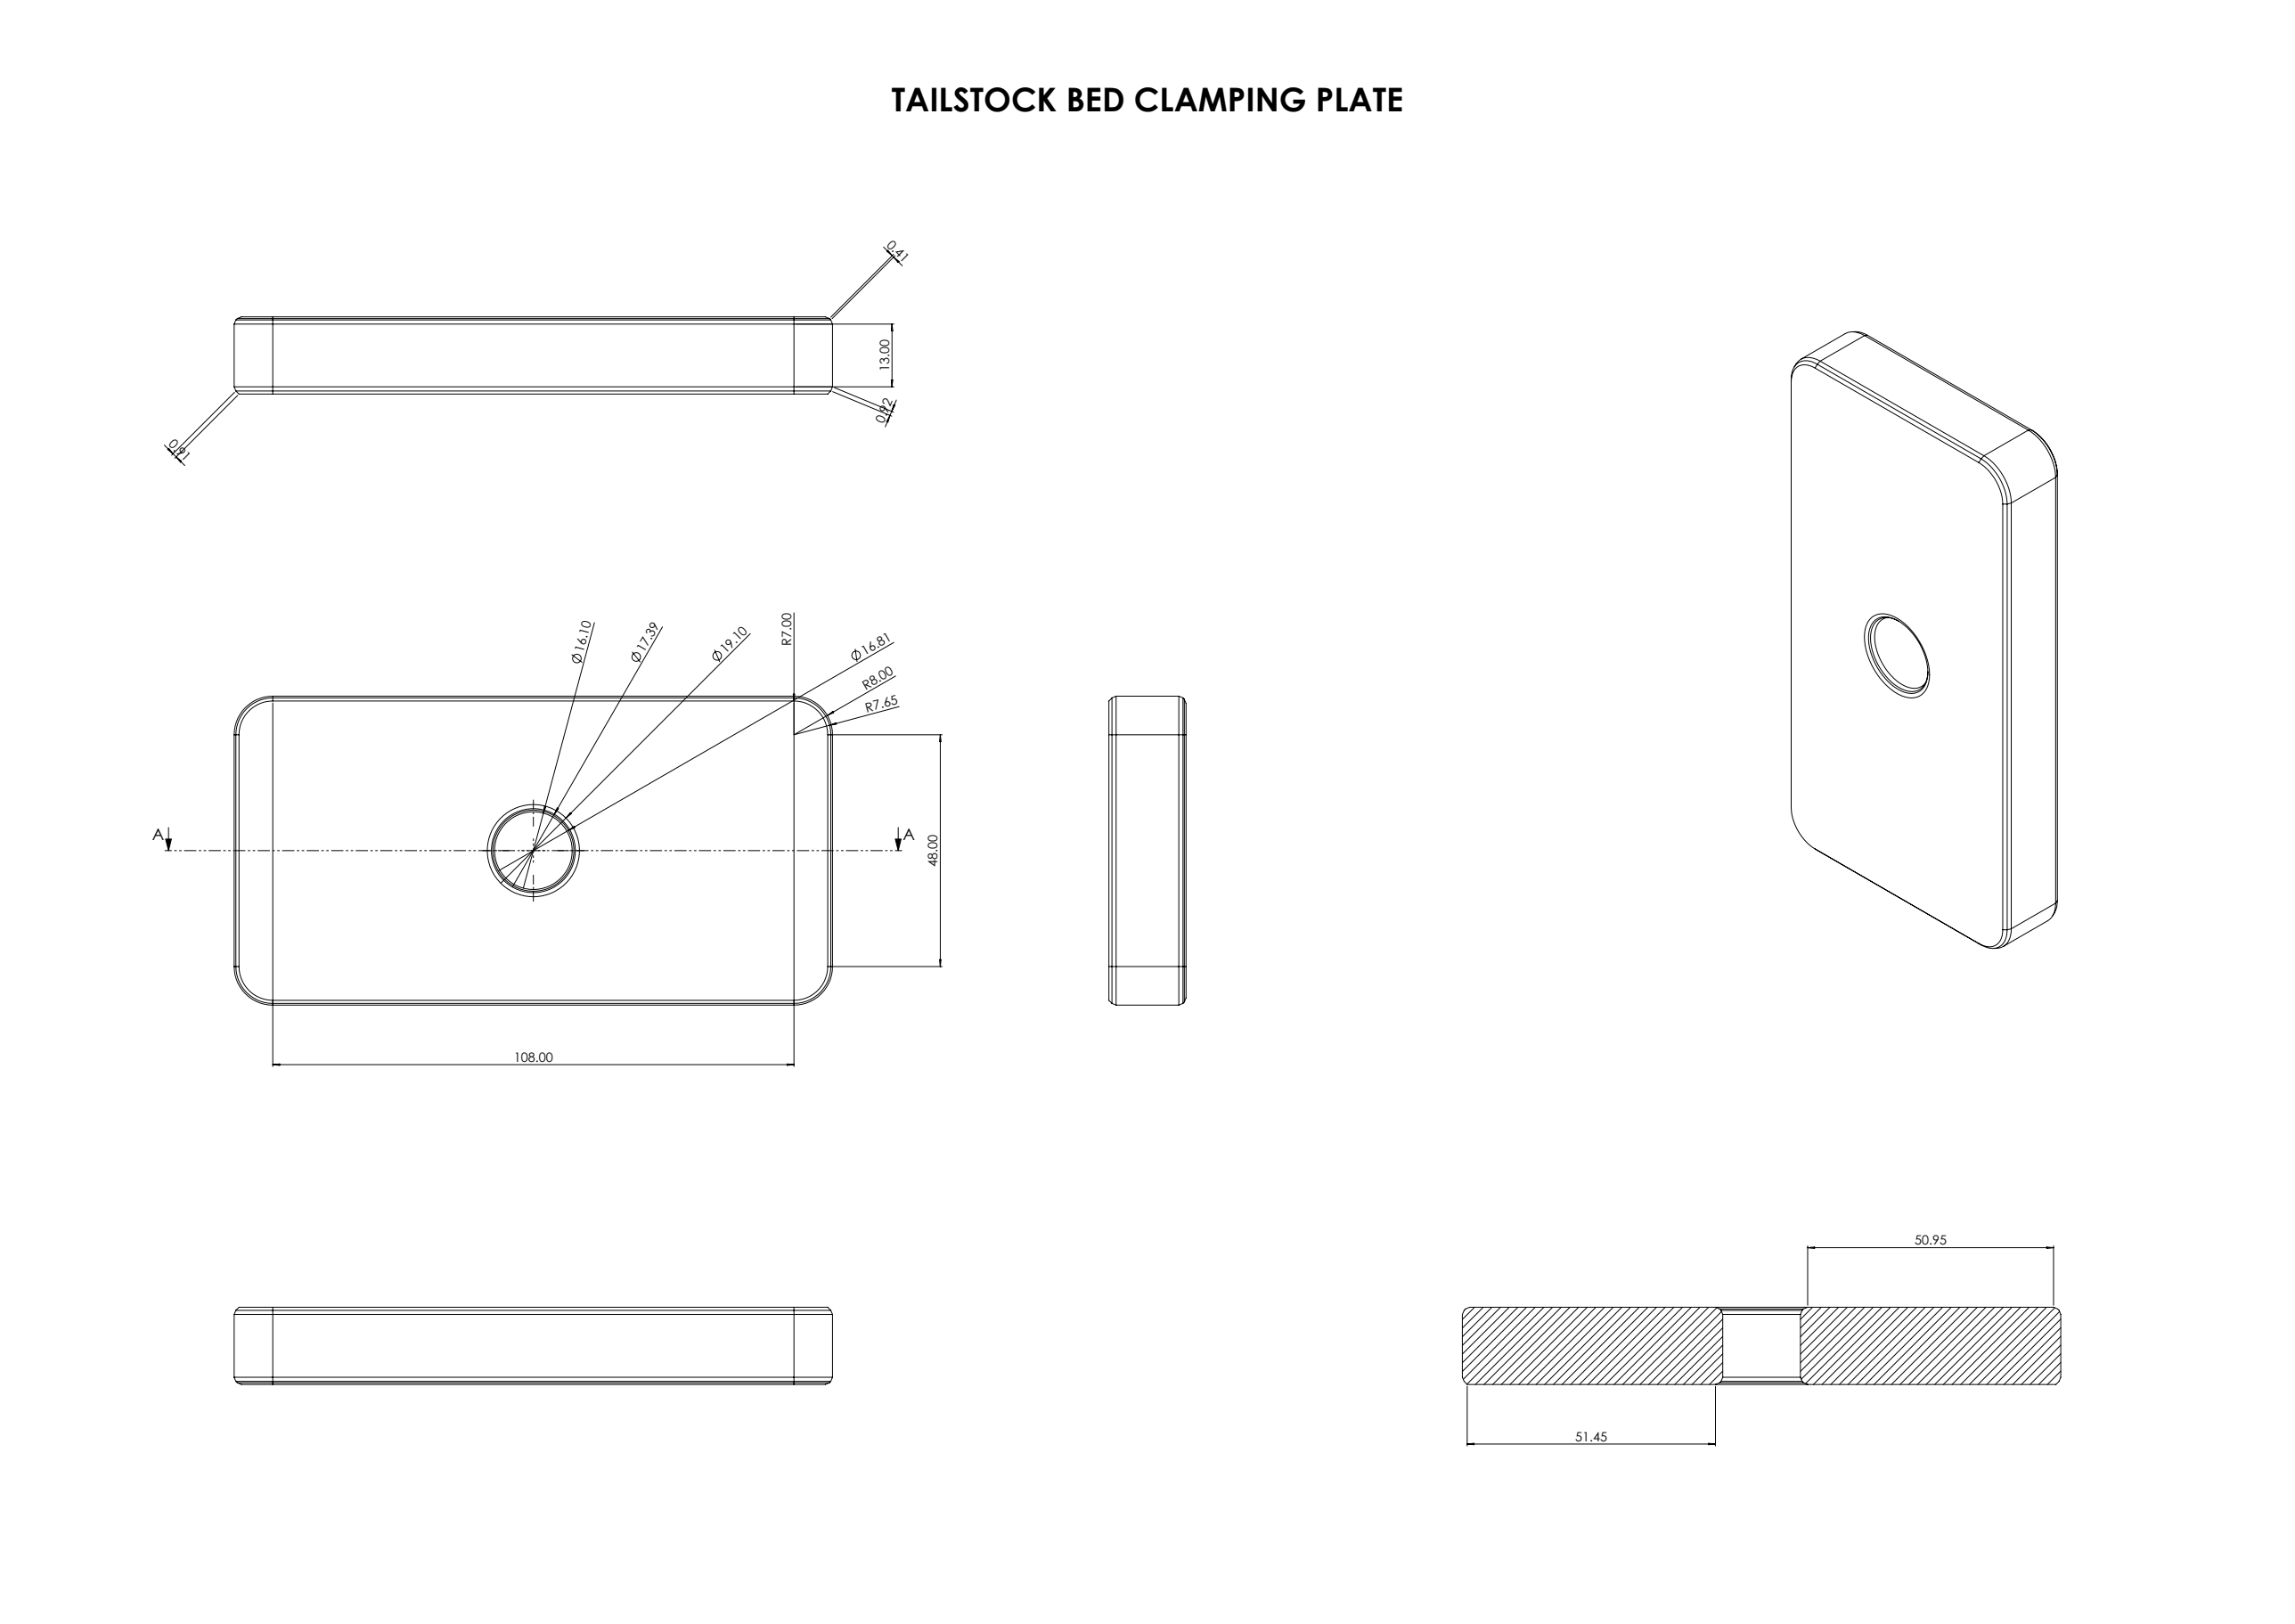
ISO-10303-21;
HEADER;
/* Generated by software containing ST-Developer
 * from STEP Tools, Inc. (www.steptools.com) 
 */

FILE_DESCRIPTION(
/* description */ (''),
/* implementation_level */ '2;1');

FILE_NAME(
/* name */ '18_Tailstock_Bed_Clamping_Plate.step',
/* time_stamp */ '2026-10-26T03:50:32-07:00',
/* author */ (''),
/* organization */ (''),
/* preprocessor_version */ 'ST-DEVELOPER v20.2',
/* originating_system */ 'Autodesk Translation Framework v15.15.0.0',
/* authorisation */ '');

FILE_SCHEMA (('AUTOMOTIVE_DESIGN { 1 0 10303 214 3 1 1 }'));
ENDSEC;

DATA;
#10=MECHANICAL_DESIGN_GEOMETRIC_PRESENTATION_REPRESENTATION('',(#1054),#76660);
#1014=SHAPE_REPRESENTATION_RELATIONSHIP('SRR','None',#76751,#1034);
#1034=ADVANCED_BREP_SHAPE_REPRESENTATION('',(#1074),#76655);
#1054=STYLED_ITEM('',(#76920),#1074);
#1074=MANIFOLD_SOLID_BREP('Clamping plate',#26679);
#1402=CYLINDRICAL_SURFACE('',#28444,0.805);
#1403=CYLINDRICAL_SURFACE('',#28474,0.800000000000004);
#1404=CYLINDRICAL_SURFACE('',#28477,0.799999999999997);
#1405=CYLINDRICAL_SURFACE('',#28521,0.799999999999998);
#1406=CYLINDRICAL_SURFACE('',#28523,0.800000000000004);
#1642=FACE_BOUND('',#5156,.T.);
#1643=FACE_BOUND('',#5163,.T.);
#2159=PLANE('',#28437);
#2160=PLANE('',#28452);
#2161=PLANE('',#28460);
#2162=PLANE('',#28464);
#2163=PLANE('',#28468);
#2164=PLANE('',#28472);
#2165=PLANE('',#28473);
#2166=PLANE('',#28476);
#2167=PLANE('',#28479);
#2168=PLANE('',#28481);
#2169=PLANE('',#28483);
#2170=PLANE('',#28486);
#2171=PLANE('',#28489);
#2172=PLANE('',#28492);
#2173=PLANE('',#28497);
#2174=PLANE('',#28500);
#2175=PLANE('',#28501);
#2176=PLANE('',#28503);
#2177=PLANE('',#28505);
#2178=PLANE('',#28509);
#2179=PLANE('',#28514);
#2180=PLANE('',#28516);
#2181=PLANE('',#28517);
#2182=PLANE('',#28519);
#2183=PLANE('',#28522);
#2184=PLANE('',#28524);
#3512=FACE_OUTER_BOUND('',#5153,.T.);
#3513=FACE_OUTER_BOUND('',#5154,.T.);
#3514=FACE_OUTER_BOUND('',#5155,.T.);
#3515=FACE_OUTER_BOUND('',#5157,.T.);
#3516=FACE_OUTER_BOUND('',#5158,.T.);
#3517=FACE_OUTER_BOUND('',#5159,.T.);
#3518=FACE_OUTER_BOUND('',#5160,.T.);
#3519=FACE_OUTER_BOUND('',#5161,.T.);
#3520=FACE_OUTER_BOUND('',#5162,.T.);
#3521=FACE_OUTER_BOUND('',#5164,.T.);
#3522=FACE_OUTER_BOUND('',#5165,.T.);
#3523=FACE_OUTER_BOUND('',#5166,.T.);
#3524=FACE_OUTER_BOUND('',#5167,.T.);
#3525=FACE_OUTER_BOUND('',#5168,.T.);
#3526=FACE_OUTER_BOUND('',#5169,.T.);
#3527=FACE_OUTER_BOUND('',#5170,.T.);
#3528=FACE_OUTER_BOUND('',#5171,.T.);
#3529=FACE_OUTER_BOUND('',#5172,.T.);
#3530=FACE_OUTER_BOUND('',#5173,.T.);
#3531=FACE_OUTER_BOUND('',#5174,.T.);
#3532=FACE_OUTER_BOUND('',#5175,.T.);
#3533=FACE_OUTER_BOUND('',#5176,.T.);
#3534=FACE_OUTER_BOUND('',#5177,.T.);
#3535=FACE_OUTER_BOUND('',#5178,.T.);
#3536=FACE_OUTER_BOUND('',#5179,.T.);
#3537=FACE_OUTER_BOUND('',#5180,.T.);
#3538=FACE_OUTER_BOUND('',#5181,.T.);
#3539=FACE_OUTER_BOUND('',#5182,.T.);
#3540=FACE_OUTER_BOUND('',#5183,.T.);
#3541=FACE_OUTER_BOUND('',#5184,.T.);
#3542=FACE_OUTER_BOUND('',#5185,.T.);
#3543=FACE_OUTER_BOUND('',#5186,.T.);
#3544=FACE_OUTER_BOUND('',#5187,.T.);
#3545=FACE_OUTER_BOUND('',#5188,.T.);
#3546=FACE_OUTER_BOUND('',#5189,.T.);
#3547=FACE_OUTER_BOUND('',#5190,.T.);
#3548=FACE_OUTER_BOUND('',#5191,.T.);
#3549=FACE_OUTER_BOUND('',#5192,.T.);
#3550=FACE_OUTER_BOUND('',#5193,.T.);
#3551=FACE_OUTER_BOUND('',#5194,.T.);
#3552=FACE_OUTER_BOUND('',#5195,.T.);
#3553=FACE_OUTER_BOUND('',#5196,.T.);
#3554=FACE_OUTER_BOUND('',#5197,.T.);
#3555=FACE_OUTER_BOUND('',#5198,.T.);
#3556=FACE_OUTER_BOUND('',#5199,.T.);
#3557=FACE_OUTER_BOUND('',#5200,.T.);
#3558=FACE_OUTER_BOUND('',#5201,.T.);
#3559=FACE_OUTER_BOUND('',#5202,.T.);
#3560=FACE_OUTER_BOUND('',#5203,.T.);
#3561=FACE_OUTER_BOUND('',#5204,.T.);
#3562=FACE_OUTER_BOUND('',#5205,.T.);
#3563=FACE_OUTER_BOUND('',#5206,.T.);
#3564=FACE_OUTER_BOUND('',#5207,.T.);
#3565=FACE_OUTER_BOUND('',#5208,.T.);
#3566=FACE_OUTER_BOUND('',#5209,.T.);
#3567=FACE_OUTER_BOUND('',#5210,.T.);
#3568=FACE_OUTER_BOUND('',#5211,.T.);
#5153=EDGE_LOOP('',(#22121,#22122,#22123,#22124));
#5154=EDGE_LOOP('',(#22125,#22126,#22127,#22128));
#5155=EDGE_LOOP('',(#22129,#22130,#22131,#22132,#22133,#22134,#22135,#22136));
#5156=EDGE_LOOP('',(#22137));
#5157=EDGE_LOOP('',(#22138,#22139,#22140,#22141));
#5158=EDGE_LOOP('',(#22142,#22143,#22144,#22145));
#5159=EDGE_LOOP('',(#22146,#22147,#22148,#22149));
#5160=EDGE_LOOP('',(#22150,#22151,#22152,#22153));
#5161=EDGE_LOOP('',(#22154,#22155,#22156,#22157));
#5162=EDGE_LOOP('',(#22158,#22159,#22160,#22161,#22162,#22163,#22164,#22165));
#5163=EDGE_LOOP('',(#22166));
#5164=EDGE_LOOP('',(#22167,#22168,#22169,#22170));
#5165=EDGE_LOOP('',(#22171,#22172,#22173,#22174));
#5166=EDGE_LOOP('',(#22175,#22176,#22177,#22178));
#5167=EDGE_LOOP('',(#22179,#22180,#22181,#22182));
#5168=EDGE_LOOP('',(#22183,#22184,#22185,#22186));
#5169=EDGE_LOOP('',(#22187,#22188,#22189,#22190));
#5170=EDGE_LOOP('',(#22191,#22192,#22193,#22194));
#5171=EDGE_LOOP('',(#22195,#22196,#22197,#22198));
#5172=EDGE_LOOP('',(#22199,#22200,#22201,#22202));
#5173=EDGE_LOOP('',(#22203,#22204,#22205,#22206));
#5174=EDGE_LOOP('',(#22207,#22208,#22209,#22210));
#5175=EDGE_LOOP('',(#22211,#22212,#22213,#22214));
#5176=EDGE_LOOP('',(#22215,#22216,#22217,#22218));
#5177=EDGE_LOOP('',(#22219,#22220,#22221,#22222));
#5178=EDGE_LOOP('',(#22223,#22224,#22225,#22226));
#5179=EDGE_LOOP('',(#22227,#22228,#22229,#22230));
#5180=EDGE_LOOP('',(#22231,#22232,#22233,#22234));
#5181=EDGE_LOOP('',(#22235,#22236,#22237,#22238));
#5182=EDGE_LOOP('',(#22239,#22240,#22241,#22242));
#5183=EDGE_LOOP('',(#22243,#22244,#22245,#22246));
#5184=EDGE_LOOP('',(#22247,#22248,#22249,#22250));
#5185=EDGE_LOOP('',(#22251,#22252,#22253,#22254));
#5186=EDGE_LOOP('',(#22255,#22256,#22257,#22258));
#5187=EDGE_LOOP('',(#22259,#22260,#22261,#22262));
#5188=EDGE_LOOP('',(#22263,#22264,#22265,#22266));
#5189=EDGE_LOOP('',(#22267,#22268,#22269,#22270));
#5190=EDGE_LOOP('',(#22271,#22272,#22273,#22274));
#5191=EDGE_LOOP('',(#22275,#22276,#22277,#22278));
#5192=EDGE_LOOP('',(#22279,#22280,#22281,#22282));
#5193=EDGE_LOOP('',(#22283,#22284,#22285,#22286));
#5194=EDGE_LOOP('',(#22287,#22288,#22289,#22290));
#5195=EDGE_LOOP('',(#22291,#22292,#22293,#22294));
#5196=EDGE_LOOP('',(#22295,#22296,#22297,#22298));
#5197=EDGE_LOOP('',(#22299,#22300,#22301,#22302));
#5198=EDGE_LOOP('',(#22303,#22304,#22305,#22306));
#5199=EDGE_LOOP('',(#22307,#22308,#22309,#22310));
#5200=EDGE_LOOP('',(#22311,#22312,#22313,#22314));
#5201=EDGE_LOOP('',(#22315,#22316,#22317,#22318));
#5202=EDGE_LOOP('',(#22319,#22320,#22321,#22322));
#5203=EDGE_LOOP('',(#22323,#22324,#22325,#22326));
#5204=EDGE_LOOP('',(#22327,#22328,#22329,#22330));
#5205=EDGE_LOOP('',(#22331,#22332,#22333,#22334));
#5206=EDGE_LOOP('',(#22335,#22336,#22337,#22338));
#5207=EDGE_LOOP('',(#22339,#22340,#22341,#22342));
#5208=EDGE_LOOP('',(#22343,#22344,#22345,#22346));
#5209=EDGE_LOOP('',(#22347,#22348,#22349,#22350));
#5210=EDGE_LOOP('',(#22351,#22352,#22353,#22354));
#5211=EDGE_LOOP('',(#22355,#22356,#22357,#22358));
#6269=CIRCLE('',#28433,0.869644660940672);
#6270=CIRCLE('',#28434,0.955000000000001);
#6271=CIRCLE('',#28436,0.840355339059329);
#6272=CIRCLE('',#28438,0.700000000000004);
#6273=CIRCLE('',#28439,0.699999999999995);
#6274=CIRCLE('',#28440,0.699999999999994);
#6275=CIRCLE('',#28441,0.700000000000004);
#6276=CIRCLE('',#28443,0.805);
#6277=CIRCLE('',#28445,0.805);
#6278=CIRCLE('',#28447,0.840355339059329);
#6279=CIRCLE('',#28449,0.869644660940672);
#6280=CIRCLE('',#28451,0.955000000000001);
#6281=CIRCLE('',#28453,0.649999999999999);
#6282=CIRCLE('',#28454,0.649999999999992);
#6283=CIRCLE('',#28455,0.649999999999993);
#6284=CIRCLE('',#28456,0.650000000000003);
#6285=CIRCLE('',#28458,0.764644660940668);
#6286=CIRCLE('',#28459,0.799999999999997);
#6287=CIRCLE('',#28462,0.764644660940679);
#6288=CIRCLE('',#28463,0.800000000000004);
#6289=CIRCLE('',#28466,0.764644660940679);
#6290=CIRCLE('',#28467,0.800000000000004);
#6291=CIRCLE('',#28470,0.764644660940672);
#6292=CIRCLE('',#28471,0.799999999999998);
#6293=CIRCLE('',#28475,0.800000000000004);
#6294=CIRCLE('',#28478,0.799999999999997);
#6295=CIRCLE('',#28485,0.735355339059332);
#6296=CIRCLE('',#28488,0.735355339059321);
#6297=CIRCLE('',#28491,0.735355339059318);
#6298=CIRCLE('',#28494,0.73535533905933);
#6299=CIRCLE('',#28496,0.764644660940668);
#6300=CIRCLE('',#28499,0.764644660940678);
#6301=CIRCLE('',#28507,0.764644660940672);
#6302=CIRCLE('',#28508,0.799999999999998);
#6303=CIRCLE('',#28511,0.764644660940679);
#6304=CIRCLE('',#28512,0.800000000000004);
#7959=LINE('',#63243,#10115);
#7960=LINE('',#63247,#10116);
#7961=LINE('',#63252,#10117);
#7962=LINE('',#63256,#10118);
#7963=LINE('',#63260,#10119);
#7964=LINE('',#63264,#10120);
#7965=LINE('',#63268,#10121);
#7966=LINE('',#63273,#10122);
#7967=LINE('',#63277,#10123);
#7968=LINE('',#63281,#10124);
#7969=LINE('',#63284,#10125);
#7970=LINE('',#63289,#10126);
#7971=LINE('',#63293,#10127);
#7972=LINE('',#63297,#10128);
#7973=LINE('',#63301,#10129);
#7974=LINE('',#63306,#10130);
#7975=LINE('',#63310,#10131);
#7976=LINE('',#63315,#10132);
#7977=LINE('',#63316,#10133);
#7978=LINE('',#63317,#10134);
#7979=LINE('',#63321,#10135);
#7980=LINE('',#63327,#10136);
#7981=LINE('',#63328,#10137);
#7982=LINE('',#63329,#10138);
#7983=LINE('',#63333,#10139);
#7984=LINE('',#63339,#10140);
#7985=LINE('',#63340,#10141);
#7986=LINE('',#63341,#10142);
#7987=LINE('',#63345,#10143);
#7988=LINE('',#63349,#10144);
#7989=LINE('',#63350,#10145);
#7990=LINE('',#63353,#10146);
#7991=LINE('',#63355,#10147);
#7992=LINE('',#63356,#10148);
#7993=LINE('',#63359,#10149);
#7994=LINE('',#63363,#10150);
#7995=LINE('',#63364,#10151);
#7996=LINE('',#63367,#10152);
#7997=LINE('',#63370,#10153);
#7998=LINE('',#63371,#10154);
#7999=LINE('',#63373,#10155);
#8000=LINE('',#63375,#10156);
#8001=LINE('',#63377,#10157);
#8002=LINE('',#63380,#10158);
#8003=LINE('',#63382,#10159);
#8004=LINE('',#63383,#10160);
#8005=LINE('',#63386,#10161);
#8006=LINE('',#63390,#10162);
#8007=LINE('',#63391,#10163);
#8008=LINE('',#63394,#10164);
#8009=LINE('',#63398,#10165);
#8010=LINE('',#63399,#10166);
#8011=LINE('',#63402,#10167);
#8012=LINE('',#63406,#10168);
#8013=LINE('',#63407,#10169);
#8014=LINE('',#63412,#10170);
#8015=LINE('',#63415,#10171);
#8016=LINE('',#63418,#10172);
#8017=LINE('',#63419,#10173);
#8018=LINE('',#63422,#10174);
#8019=LINE('',#63426,#10175);
#8020=LINE('',#63427,#10176);
#8021=LINE('',#63429,#10177);
#8022=LINE('',#63430,#10178);
#8023=LINE('',#63432,#10179);
#8024=LINE('',#63434,#10180);
#8025=LINE('',#63436,#10181);
#8026=LINE('',#63440,#10182);
#8027=LINE('',#63441,#10183);
#8028=LINE('',#63442,#10184);
#8029=LINE('',#63446,#10185);
#8030=LINE('',#63452,#10186);
#8031=LINE('',#63453,#10187);
#8032=LINE('',#63454,#10188);
#8033=LINE('',#63459,#10189);
#8034=LINE('',#63460,#10190);
#8035=LINE('',#63462,#10191);
#8036=LINE('',#63466,#10192);
#8037=LINE('',#63467,#10193);
#8038=LINE('',#63470,#10194);
#8039=LINE('',#63473,#10195);
#8040=LINE('',#63474,#10196);
#8041=LINE('',#63476,#10197);
#10115=VECTOR('',#33770,0.912322330470337);
#10116=VECTOR('',#33775,0.855);
#10117=VECTOR('',#33780,1.);
#10118=VECTOR('',#33783,1.);
#10119=VECTOR('',#33786,1.);
#10120=VECTOR('',#33789,1.);
#10121=VECTOR('',#33794,0.822677669529664);
#10122=VECTOR('',#33801,0.805);
#10123=VECTOR('',#33806,0.822677669529664);
#10124=VECTOR('',#33811,0.855000000000001);
#10125=VECTOR('',#33814,0.912322330470337);
#10126=VECTOR('',#33819,1.);
#10127=VECTOR('',#33822,1.);
#10128=VECTOR('',#33825,1.);
#10129=VECTOR('',#33828,1.);
#10130=VECTOR('',#33833,1.);
#10131=VECTOR('',#33836,1.);
#10132=VECTOR('',#33841,1.);
#10133=VECTOR('',#33842,1.);
#10134=VECTOR('',#33843,1.);
#10135=VECTOR('',#33846,1.);
#10136=VECTOR('',#33853,1.);
#10137=VECTOR('',#33854,1.);
#10138=VECTOR('',#33855,1.);
#10139=VECTOR('',#33858,1.);
#10140=VECTOR('',#33865,1.);
#10141=VECTOR('',#33866,1.);
#10142=VECTOR('',#33867,1.);
#10143=VECTOR('',#33870,1.);
#10144=VECTOR('',#33877,1.);
#10145=VECTOR('',#33878,1.);
#10146=VECTOR('',#33881,1.);
#10147=VECTOR('',#33882,1.);
#10148=VECTOR('',#33883,1.);
#10149=VECTOR('',#33886,1.);
#10150=VECTOR('',#33891,1.);
#10151=VECTOR('',#33892,1.);
#10152=VECTOR('',#33895,1.);
#10153=VECTOR('',#33900,1.);
#10154=VECTOR('',#33901,1.);
#10155=VECTOR('',#33904,1.);
#10156=VECTOR('',#33907,1.);
#10157=VECTOR('',#33910,1.);
#10158=VECTOR('',#33913,1.);
#10159=VECTOR('',#33914,1.);
#10160=VECTOR('',#33915,1.);
#10161=VECTOR('',#33918,1.);
#10162=VECTOR('',#33923,1.);
#10163=VECTOR('',#33924,1.);
#10164=VECTOR('',#33927,1.);
#10165=VECTOR('',#33932,1.);
#10166=VECTOR('',#33933,1.);
#10167=VECTOR('',#33936,1.);
#10168=VECTOR('',#33941,1.);
#10169=VECTOR('',#33942,1.);
#10170=VECTOR('',#33949,1.);
#10171=VECTOR('',#33952,1.);
#10172=VECTOR('',#33955,1.);
#10173=VECTOR('',#33956,1.);
#10174=VECTOR('',#33959,1.);
#10175=VECTOR('',#33964,1.);
#10176=VECTOR('',#33965,1.);
#10177=VECTOR('',#33968,1.);
#10178=VECTOR('',#33969,1.);
#10179=VECTOR('',#33972,1.);
#10180=VECTOR('',#33975,1.);
#10181=VECTOR('',#33978,1.);
#10182=VECTOR('',#33981,1.);
#10183=VECTOR('',#33982,1.);
#10184=VECTOR('',#33983,1.);
#10185=VECTOR('',#33986,1.);
#10186=VECTOR('',#33993,1.);
#10187=VECTOR('',#33994,1.);
#10188=VECTOR('',#33995,1.);
#10189=VECTOR('',#34004,1.);
#10190=VECTOR('',#34005,1.);
#10191=VECTOR('',#34008,1.);
#10192=VECTOR('',#34015,1.);
#10193=VECTOR('',#34016,1.);
#10194=VECTOR('',#34021,1.);
#10195=VECTOR('',#34026,1.);
#10196=VECTOR('',#34027,1.);
#10197=VECTOR('',#34030,1.);
#12457=VERTEX_POINT('',#63240);
#12458=VERTEX_POINT('',#63242);
#12459=VERTEX_POINT('',#63246);
#12460=VERTEX_POINT('',#63250);
#12461=VERTEX_POINT('',#63251);
#12462=VERTEX_POINT('',#63253);
#12463=VERTEX_POINT('',#63255);
#12464=VERTEX_POINT('',#63257);
#12465=VERTEX_POINT('',#63259);
#12466=VERTEX_POINT('',#63261);
#12467=VERTEX_POINT('',#63263);
#12468=VERTEX_POINT('',#63267);
#12469=VERTEX_POINT('',#63271);
#12470=VERTEX_POINT('',#63275);
#12471=VERTEX_POINT('',#63279);
#12472=VERTEX_POINT('',#63283);
#12473=VERTEX_POINT('',#63287);
#12474=VERTEX_POINT('',#63288);
#12475=VERTEX_POINT('',#63290);
#12476=VERTEX_POINT('',#63292);
#12477=VERTEX_POINT('',#63294);
#12478=VERTEX_POINT('',#63296);
#12479=VERTEX_POINT('',#63298);
#12480=VERTEX_POINT('',#63300);
#12481=VERTEX_POINT('',#63304);
#12482=VERTEX_POINT('',#63305);
#12483=VERTEX_POINT('',#63307);
#12484=VERTEX_POINT('',#63309);
#12485=VERTEX_POINT('',#63313);
#12486=VERTEX_POINT('',#63314);
#12487=VERTEX_POINT('',#63319);
#12488=VERTEX_POINT('',#63320);
#12489=VERTEX_POINT('',#63325);
#12490=VERTEX_POINT('',#63326);
#12491=VERTEX_POINT('',#63331);
#12492=VERTEX_POINT('',#63332);
#12493=VERTEX_POINT('',#63337);
#12494=VERTEX_POINT('',#63338);
#12495=VERTEX_POINT('',#63343);
#12496=VERTEX_POINT('',#63344);
#12497=VERTEX_POINT('',#63352);
#12498=VERTEX_POINT('',#63354);
#12499=VERTEX_POINT('',#63358);
#12500=VERTEX_POINT('',#63362);
#12501=VERTEX_POINT('',#63366);
#12502=VERTEX_POINT('',#63379);
#12503=VERTEX_POINT('',#63381);
#12504=VERTEX_POINT('',#63385);
#12505=VERTEX_POINT('',#63389);
#12506=VERTEX_POINT('',#63393);
#12507=VERTEX_POINT('',#63397);
#12508=VERTEX_POINT('',#63401);
#12509=VERTEX_POINT('',#63405);
#12510=VERTEX_POINT('',#63411);
#12511=VERTEX_POINT('',#63413);
#12512=VERTEX_POINT('',#63417);
#12513=VERTEX_POINT('',#63421);
#12514=VERTEX_POINT('',#63425);
#12515=VERTEX_POINT('',#63438);
#12516=VERTEX_POINT('',#63439);
#12517=VERTEX_POINT('',#63444);
#12518=VERTEX_POINT('',#63445);
#12519=VERTEX_POINT('',#63450);
#12520=VERTEX_POINT('',#63451);
#15783=EDGE_CURVE('',#12457,#12457,#6269,.T.);
#15784=EDGE_CURVE('',#12457,#12458,#7959,.T.);
#15785=EDGE_CURVE('',#12458,#12458,#6270,.T.);
#15786=EDGE_CURVE('',#12457,#12459,#7960,.T.);
#15787=EDGE_CURVE('',#12459,#12459,#6271,.T.);
#15788=EDGE_CURVE('',#12460,#12461,#7961,.T.);
#15789=EDGE_CURVE('',#12462,#12460,#6272,.T.);
#15790=EDGE_CURVE('',#12463,#12462,#7962,.T.);
#15791=EDGE_CURVE('',#12464,#12463,#6273,.T.);
#15792=EDGE_CURVE('',#12465,#12464,#7963,.T.);
#15793=EDGE_CURVE('',#12466,#12465,#6274,.T.);
#15794=EDGE_CURVE('',#12467,#12466,#7964,.T.);
#15795=EDGE_CURVE('',#12461,#12467,#6275,.T.);
#15796=EDGE_CURVE('',#12459,#12468,#7965,.T.);
#15797=EDGE_CURVE('',#12468,#12468,#6276,.T.);
#15798=EDGE_CURVE('',#12469,#12469,#6277,.T.);
#15799=EDGE_CURVE('',#12469,#12468,#7966,.T.);
#15800=EDGE_CURVE('',#12470,#12470,#6278,.T.);
#15801=EDGE_CURVE('',#12470,#12469,#7967,.T.);
#15802=EDGE_CURVE('',#12471,#12471,#6279,.T.);
#15803=EDGE_CURVE('',#12471,#12470,#7968,.T.);
#15804=EDGE_CURVE('',#12471,#12472,#7969,.T.);
#15805=EDGE_CURVE('',#12472,#12472,#6280,.T.);
#15806=EDGE_CURVE('',#12473,#12474,#7970,.T.);
#15807=EDGE_CURVE('',#12475,#12473,#6281,.T.);
#15808=EDGE_CURVE('',#12476,#12475,#7971,.T.);
#15809=EDGE_CURVE('',#12477,#12476,#6282,.T.);
#15810=EDGE_CURVE('',#12478,#12477,#7972,.T.);
#15811=EDGE_CURVE('',#12479,#12478,#6283,.T.);
#15812=EDGE_CURVE('',#12480,#12479,#7973,.T.);
#15813=EDGE_CURVE('',#12474,#12480,#6284,.T.);
#15814=EDGE_CURVE('',#12481,#12482,#7974,.T.);
#15815=EDGE_CURVE('',#12482,#12483,#6285,.T.);
#15816=EDGE_CURVE('',#12483,#12484,#7975,.T.);
#15817=EDGE_CURVE('',#12484,#12481,#6286,.T.);
#15818=EDGE_CURVE('',#12485,#12486,#7976,.T.);
#15819=EDGE_CURVE('',#12486,#12482,#7977,.T.);
#15820=EDGE_CURVE('',#12481,#12485,#7978,.T.);
#15821=EDGE_CURVE('',#12487,#12488,#7979,.T.);
#15822=EDGE_CURVE('',#12488,#12486,#6287,.T.);
#15823=EDGE_CURVE('',#12485,#12487,#6288,.T.);
#15824=EDGE_CURVE('',#12489,#12490,#7980,.T.);
#15825=EDGE_CURVE('',#12490,#12488,#7981,.T.);
#15826=EDGE_CURVE('',#12487,#12489,#7982,.T.);
#15827=EDGE_CURVE('',#12491,#12492,#7983,.T.);
#15828=EDGE_CURVE('',#12492,#12490,#6289,.T.);
#15829=EDGE_CURVE('',#12489,#12491,#6290,.T.);
#15830=EDGE_CURVE('',#12493,#12494,#7984,.T.);
#15831=EDGE_CURVE('',#12494,#12492,#7985,.T.);
#15832=EDGE_CURVE('',#12491,#12493,#7986,.T.);
#15833=EDGE_CURVE('',#12495,#12496,#7987,.T.);
#15834=EDGE_CURVE('',#12496,#12494,#6291,.T.);
#15835=EDGE_CURVE('',#12493,#12495,#6292,.T.);
#15836=EDGE_CURVE('',#12483,#12496,#7988,.T.);
#15837=EDGE_CURVE('',#12495,#12484,#7989,.T.);
#15838=EDGE_CURVE('',#12497,#12487,#7990,.T.);
#15839=EDGE_CURVE('',#12498,#12497,#7991,.T.);
#15840=EDGE_CURVE('',#12498,#12489,#7992,.T.);
#15841=EDGE_CURVE('',#12499,#12485,#7993,.T.);
#15842=EDGE_CURVE('',#12497,#12499,#6293,.T.);
#15843=EDGE_CURVE('',#12500,#12481,#7994,.T.);
#15844=EDGE_CURVE('',#12499,#12500,#7995,.T.);
#15845=EDGE_CURVE('',#12501,#12484,#7996,.T.);
#15846=EDGE_CURVE('',#12500,#12501,#6294,.T.);
#15847=EDGE_CURVE('',#12494,#12463,#7997,.T.);
#15848=EDGE_CURVE('',#12492,#12462,#7998,.T.);
#15849=EDGE_CURVE('',#12496,#12464,#7999,.T.);
#15850=EDGE_CURVE('',#12483,#12465,#8000,.T.);
#15851=EDGE_CURVE('',#12482,#12466,#8001,.T.);
#15852=EDGE_CURVE('',#12474,#12502,#8002,.T.);
#15853=EDGE_CURVE('',#12502,#12503,#8003,.T.);
#15854=EDGE_CURVE('',#12503,#12473,#8004,.T.);
#15855=EDGE_CURVE('',#12480,#12504,#8005,.T.);
#15856=EDGE_CURVE('',#12504,#12502,#6295,.T.);
#15857=EDGE_CURVE('',#12479,#12505,#8006,.T.);
#15858=EDGE_CURVE('',#12505,#12504,#8007,.T.);
#15859=EDGE_CURVE('',#12478,#12506,#8008,.T.);
#15860=EDGE_CURVE('',#12506,#12505,#6296,.T.);
#15861=EDGE_CURVE('',#12477,#12507,#8009,.T.);
#15862=EDGE_CURVE('',#12507,#12506,#8010,.T.);
#15863=EDGE_CURVE('',#12476,#12508,#8011,.T.);
#15864=EDGE_CURVE('',#12508,#12507,#6297,.T.);
#15865=EDGE_CURVE('',#12475,#12509,#8012,.T.);
#15866=EDGE_CURVE('',#12509,#12508,#8013,.T.);
#15867=EDGE_CURVE('',#12503,#12509,#6298,.T.);
#15868=EDGE_CURVE('',#12508,#12510,#8014,.T.);
#15869=EDGE_CURVE('',#12511,#12510,#6299,.T.);
#15870=EDGE_CURVE('',#12507,#12511,#8015,.T.);
#15871=EDGE_CURVE('',#12509,#12512,#8016,.T.);
#15872=EDGE_CURVE('',#12510,#12512,#8017,.T.);
#15873=EDGE_CURVE('',#12513,#12503,#8018,.T.);
#15874=EDGE_CURVE('',#12512,#12513,#6300,.T.);
#15875=EDGE_CURVE('',#12502,#12514,#8019,.T.);
#15876=EDGE_CURVE('',#12513,#12514,#8020,.T.);
#15877=EDGE_CURVE('',#12497,#12513,#8021,.T.);
#15878=EDGE_CURVE('',#12514,#12498,#8022,.T.);
#15879=EDGE_CURVE('',#12499,#12512,#8023,.T.);
#15880=EDGE_CURVE('',#12500,#12510,#8024,.T.);
#15881=EDGE_CURVE('',#12501,#12511,#8025,.T.);
#15882=EDGE_CURVE('',#12515,#12516,#8026,.T.);
#15883=EDGE_CURVE('',#12516,#12511,#8027,.T.);
#15884=EDGE_CURVE('',#12501,#12515,#8028,.T.);
#15885=EDGE_CURVE('',#12517,#12518,#8029,.T.);
#15886=EDGE_CURVE('',#12518,#12516,#6301,.T.);
#15887=EDGE_CURVE('',#12515,#12517,#6302,.T.);
#15888=EDGE_CURVE('',#12519,#12520,#8030,.T.);
#15889=EDGE_CURVE('',#12520,#12518,#8031,.T.);
#15890=EDGE_CURVE('',#12517,#12519,#8032,.T.);
#15891=EDGE_CURVE('',#12514,#12520,#6303,.T.);
#15892=EDGE_CURVE('',#12519,#12498,#6304,.T.);
#15893=EDGE_CURVE('',#12506,#12516,#8033,.T.);
#15894=EDGE_CURVE('',#12505,#12518,#8034,.T.);
#15895=EDGE_CURVE('',#12504,#12520,#8035,.T.);
#15896=EDGE_CURVE('',#12490,#12460,#8036,.T.);
#15897=EDGE_CURVE('',#12461,#12488,#8037,.T.);
#15898=EDGE_CURVE('',#12486,#12467,#8038,.T.);
#15899=EDGE_CURVE('',#12517,#12493,#8039,.T.);
#15900=EDGE_CURVE('',#12515,#12495,#8040,.T.);
#15901=EDGE_CURVE('',#12519,#12491,#8041,.T.);
#22121=ORIENTED_EDGE('',*,*,#15783,.T.);
#22122=ORIENTED_EDGE('',*,*,#15784,.T.);
#22123=ORIENTED_EDGE('',*,*,#15785,.T.);
#22124=ORIENTED_EDGE('',*,*,#15784,.F.);
#22125=ORIENTED_EDGE('',*,*,#15783,.F.);
#22126=ORIENTED_EDGE('',*,*,#15786,.T.);
#22127=ORIENTED_EDGE('',*,*,#15787,.F.);
#22128=ORIENTED_EDGE('',*,*,#15786,.F.);
#22129=ORIENTED_EDGE('',*,*,#15788,.F.);
#22130=ORIENTED_EDGE('',*,*,#15789,.F.);
#22131=ORIENTED_EDGE('',*,*,#15790,.F.);
#22132=ORIENTED_EDGE('',*,*,#15791,.F.);
#22133=ORIENTED_EDGE('',*,*,#15792,.F.);
#22134=ORIENTED_EDGE('',*,*,#15793,.F.);
#22135=ORIENTED_EDGE('',*,*,#15794,.F.);
#22136=ORIENTED_EDGE('',*,*,#15795,.F.);
#22137=ORIENTED_EDGE('',*,*,#15785,.F.);
#22138=ORIENTED_EDGE('',*,*,#15787,.T.);
#22139=ORIENTED_EDGE('',*,*,#15796,.T.);
#22140=ORIENTED_EDGE('',*,*,#15797,.T.);
#22141=ORIENTED_EDGE('',*,*,#15796,.F.);
#22142=ORIENTED_EDGE('',*,*,#15798,.F.);
#22143=ORIENTED_EDGE('',*,*,#15799,.T.);
#22144=ORIENTED_EDGE('',*,*,#15797,.F.);
#22145=ORIENTED_EDGE('',*,*,#15799,.F.);
#22146=ORIENTED_EDGE('',*,*,#15800,.T.);
#22147=ORIENTED_EDGE('',*,*,#15801,.T.);
#22148=ORIENTED_EDGE('',*,*,#15798,.T.);
#22149=ORIENTED_EDGE('',*,*,#15801,.F.);
#22150=ORIENTED_EDGE('',*,*,#15802,.F.);
#22151=ORIENTED_EDGE('',*,*,#15803,.T.);
#22152=ORIENTED_EDGE('',*,*,#15800,.F.);
#22153=ORIENTED_EDGE('',*,*,#15803,.F.);
#22154=ORIENTED_EDGE('',*,*,#15802,.T.);
#22155=ORIENTED_EDGE('',*,*,#15804,.T.);
#22156=ORIENTED_EDGE('',*,*,#15805,.T.);
#22157=ORIENTED_EDGE('',*,*,#15804,.F.);
#22158=ORIENTED_EDGE('',*,*,#15806,.F.);
#22159=ORIENTED_EDGE('',*,*,#15807,.F.);
#22160=ORIENTED_EDGE('',*,*,#15808,.F.);
#22161=ORIENTED_EDGE('',*,*,#15809,.F.);
#22162=ORIENTED_EDGE('',*,*,#15810,.F.);
#22163=ORIENTED_EDGE('',*,*,#15811,.F.);
#22164=ORIENTED_EDGE('',*,*,#15812,.F.);
#22165=ORIENTED_EDGE('',*,*,#15813,.F.);
#22166=ORIENTED_EDGE('',*,*,#15805,.F.);
#22167=ORIENTED_EDGE('',*,*,#15814,.T.);
#22168=ORIENTED_EDGE('',*,*,#15815,.T.);
#22169=ORIENTED_EDGE('',*,*,#15816,.T.);
#22170=ORIENTED_EDGE('',*,*,#15817,.T.);
#22171=ORIENTED_EDGE('',*,*,#15818,.T.);
#22172=ORIENTED_EDGE('',*,*,#15819,.T.);
#22173=ORIENTED_EDGE('',*,*,#15814,.F.);
#22174=ORIENTED_EDGE('',*,*,#15820,.T.);
#22175=ORIENTED_EDGE('',*,*,#15821,.T.);
#22176=ORIENTED_EDGE('',*,*,#15822,.T.);
#22177=ORIENTED_EDGE('',*,*,#15818,.F.);
#22178=ORIENTED_EDGE('',*,*,#15823,.T.);
#22179=ORIENTED_EDGE('',*,*,#15824,.T.);
#22180=ORIENTED_EDGE('',*,*,#15825,.T.);
#22181=ORIENTED_EDGE('',*,*,#15821,.F.);
#22182=ORIENTED_EDGE('',*,*,#15826,.T.);
#22183=ORIENTED_EDGE('',*,*,#15827,.T.);
#22184=ORIENTED_EDGE('',*,*,#15828,.T.);
#22185=ORIENTED_EDGE('',*,*,#15824,.F.);
#22186=ORIENTED_EDGE('',*,*,#15829,.T.);
#22187=ORIENTED_EDGE('',*,*,#15830,.T.);
#22188=ORIENTED_EDGE('',*,*,#15831,.T.);
#22189=ORIENTED_EDGE('',*,*,#15827,.F.);
#22190=ORIENTED_EDGE('',*,*,#15832,.T.);
#22191=ORIENTED_EDGE('',*,*,#15833,.T.);
#22192=ORIENTED_EDGE('',*,*,#15834,.T.);
#22193=ORIENTED_EDGE('',*,*,#15830,.F.);
#22194=ORIENTED_EDGE('',*,*,#15835,.T.);
#22195=ORIENTED_EDGE('',*,*,#15816,.F.);
#22196=ORIENTED_EDGE('',*,*,#15836,.T.);
#22197=ORIENTED_EDGE('',*,*,#15833,.F.);
#22198=ORIENTED_EDGE('',*,*,#15837,.T.);
#22199=ORIENTED_EDGE('',*,*,#15826,.F.);
#22200=ORIENTED_EDGE('',*,*,#15838,.F.);
#22201=ORIENTED_EDGE('',*,*,#15839,.F.);
#22202=ORIENTED_EDGE('',*,*,#15840,.T.);
#22203=ORIENTED_EDGE('',*,*,#15823,.F.);
#22204=ORIENTED_EDGE('',*,*,#15841,.F.);
#22205=ORIENTED_EDGE('',*,*,#15842,.F.);
#22206=ORIENTED_EDGE('',*,*,#15838,.T.);
#22207=ORIENTED_EDGE('',*,*,#15820,.F.);
#22208=ORIENTED_EDGE('',*,*,#15843,.F.);
#22209=ORIENTED_EDGE('',*,*,#15844,.F.);
#22210=ORIENTED_EDGE('',*,*,#15841,.T.);
#22211=ORIENTED_EDGE('',*,*,#15817,.F.);
#22212=ORIENTED_EDGE('',*,*,#15845,.F.);
#22213=ORIENTED_EDGE('',*,*,#15846,.F.);
#22214=ORIENTED_EDGE('',*,*,#15843,.T.);
#22215=ORIENTED_EDGE('',*,*,#15831,.F.);
#22216=ORIENTED_EDGE('',*,*,#15847,.T.);
#22217=ORIENTED_EDGE('',*,*,#15790,.T.);
#22218=ORIENTED_EDGE('',*,*,#15848,.F.);
#22219=ORIENTED_EDGE('',*,*,#15834,.F.);
#22220=ORIENTED_EDGE('',*,*,#15849,.T.);
#22221=ORIENTED_EDGE('',*,*,#15791,.T.);
#22222=ORIENTED_EDGE('',*,*,#15847,.F.);
#22223=ORIENTED_EDGE('',*,*,#15836,.F.);
#22224=ORIENTED_EDGE('',*,*,#15850,.T.);
#22225=ORIENTED_EDGE('',*,*,#15792,.T.);
#22226=ORIENTED_EDGE('',*,*,#15849,.F.);
#22227=ORIENTED_EDGE('',*,*,#15815,.F.);
#22228=ORIENTED_EDGE('',*,*,#15851,.T.);
#22229=ORIENTED_EDGE('',*,*,#15793,.T.);
#22230=ORIENTED_EDGE('',*,*,#15850,.F.);
#22231=ORIENTED_EDGE('',*,*,#15852,.T.);
#22232=ORIENTED_EDGE('',*,*,#15853,.T.);
#22233=ORIENTED_EDGE('',*,*,#15854,.T.);
#22234=ORIENTED_EDGE('',*,*,#15806,.T.);
#22235=ORIENTED_EDGE('',*,*,#15855,.T.);
#22236=ORIENTED_EDGE('',*,*,#15856,.T.);
#22237=ORIENTED_EDGE('',*,*,#15852,.F.);
#22238=ORIENTED_EDGE('',*,*,#15813,.T.);
#22239=ORIENTED_EDGE('',*,*,#15857,.T.);
#22240=ORIENTED_EDGE('',*,*,#15858,.T.);
#22241=ORIENTED_EDGE('',*,*,#15855,.F.);
#22242=ORIENTED_EDGE('',*,*,#15812,.T.);
#22243=ORIENTED_EDGE('',*,*,#15859,.T.);
#22244=ORIENTED_EDGE('',*,*,#15860,.T.);
#22245=ORIENTED_EDGE('',*,*,#15857,.F.);
#22246=ORIENTED_EDGE('',*,*,#15811,.T.);
#22247=ORIENTED_EDGE('',*,*,#15861,.T.);
#22248=ORIENTED_EDGE('',*,*,#15862,.T.);
#22249=ORIENTED_EDGE('',*,*,#15859,.F.);
#22250=ORIENTED_EDGE('',*,*,#15810,.T.);
#22251=ORIENTED_EDGE('',*,*,#15863,.T.);
#22252=ORIENTED_EDGE('',*,*,#15864,.T.);
#22253=ORIENTED_EDGE('',*,*,#15861,.F.);
#22254=ORIENTED_EDGE('',*,*,#15809,.T.);
#22255=ORIENTED_EDGE('',*,*,#15865,.T.);
#22256=ORIENTED_EDGE('',*,*,#15866,.T.);
#22257=ORIENTED_EDGE('',*,*,#15863,.F.);
#22258=ORIENTED_EDGE('',*,*,#15808,.T.);
#22259=ORIENTED_EDGE('',*,*,#15854,.F.);
#22260=ORIENTED_EDGE('',*,*,#15867,.T.);
#22261=ORIENTED_EDGE('',*,*,#15865,.F.);
#22262=ORIENTED_EDGE('',*,*,#15807,.T.);
#22263=ORIENTED_EDGE('',*,*,#15864,.F.);
#22264=ORIENTED_EDGE('',*,*,#15868,.T.);
#22265=ORIENTED_EDGE('',*,*,#15869,.F.);
#22266=ORIENTED_EDGE('',*,*,#15870,.F.);
#22267=ORIENTED_EDGE('',*,*,#15866,.F.);
#22268=ORIENTED_EDGE('',*,*,#15871,.T.);
#22269=ORIENTED_EDGE('',*,*,#15872,.F.);
#22270=ORIENTED_EDGE('',*,*,#15868,.F.);
#22271=ORIENTED_EDGE('',*,*,#15867,.F.);
#22272=ORIENTED_EDGE('',*,*,#15873,.F.);
#22273=ORIENTED_EDGE('',*,*,#15874,.F.);
#22274=ORIENTED_EDGE('',*,*,#15871,.F.);
#22275=ORIENTED_EDGE('',*,*,#15853,.F.);
#22276=ORIENTED_EDGE('',*,*,#15875,.T.);
#22277=ORIENTED_EDGE('',*,*,#15876,.F.);
#22278=ORIENTED_EDGE('',*,*,#15873,.T.);
#22279=ORIENTED_EDGE('',*,*,#15877,.T.);
#22280=ORIENTED_EDGE('',*,*,#15876,.T.);
#22281=ORIENTED_EDGE('',*,*,#15878,.T.);
#22282=ORIENTED_EDGE('',*,*,#15839,.T.);
#22283=ORIENTED_EDGE('',*,*,#15879,.T.);
#22284=ORIENTED_EDGE('',*,*,#15874,.T.);
#22285=ORIENTED_EDGE('',*,*,#15877,.F.);
#22286=ORIENTED_EDGE('',*,*,#15842,.T.);
#22287=ORIENTED_EDGE('',*,*,#15880,.T.);
#22288=ORIENTED_EDGE('',*,*,#15872,.T.);
#22289=ORIENTED_EDGE('',*,*,#15879,.F.);
#22290=ORIENTED_EDGE('',*,*,#15844,.T.);
#22291=ORIENTED_EDGE('',*,*,#15881,.T.);
#22292=ORIENTED_EDGE('',*,*,#15869,.T.);
#22293=ORIENTED_EDGE('',*,*,#15880,.F.);
#22294=ORIENTED_EDGE('',*,*,#15846,.T.);
#22295=ORIENTED_EDGE('',*,*,#15882,.T.);
#22296=ORIENTED_EDGE('',*,*,#15883,.T.);
#22297=ORIENTED_EDGE('',*,*,#15881,.F.);
#22298=ORIENTED_EDGE('',*,*,#15884,.T.);
#22299=ORIENTED_EDGE('',*,*,#15885,.T.);
#22300=ORIENTED_EDGE('',*,*,#15886,.T.);
#22301=ORIENTED_EDGE('',*,*,#15882,.F.);
#22302=ORIENTED_EDGE('',*,*,#15887,.T.);
#22303=ORIENTED_EDGE('',*,*,#15888,.T.);
#22304=ORIENTED_EDGE('',*,*,#15889,.T.);
#22305=ORIENTED_EDGE('',*,*,#15885,.F.);
#22306=ORIENTED_EDGE('',*,*,#15890,.T.);
#22307=ORIENTED_EDGE('',*,*,#15878,.F.);
#22308=ORIENTED_EDGE('',*,*,#15891,.T.);
#22309=ORIENTED_EDGE('',*,*,#15888,.F.);
#22310=ORIENTED_EDGE('',*,*,#15892,.T.);
#22311=ORIENTED_EDGE('',*,*,#15860,.F.);
#22312=ORIENTED_EDGE('',*,*,#15893,.T.);
#22313=ORIENTED_EDGE('',*,*,#15886,.F.);
#22314=ORIENTED_EDGE('',*,*,#15894,.F.);
#22315=ORIENTED_EDGE('',*,*,#15858,.F.);
#22316=ORIENTED_EDGE('',*,*,#15894,.T.);
#22317=ORIENTED_EDGE('',*,*,#15889,.F.);
#22318=ORIENTED_EDGE('',*,*,#15895,.F.);
#22319=ORIENTED_EDGE('',*,*,#15856,.F.);
#22320=ORIENTED_EDGE('',*,*,#15895,.T.);
#22321=ORIENTED_EDGE('',*,*,#15891,.F.);
#22322=ORIENTED_EDGE('',*,*,#15875,.F.);
#22323=ORIENTED_EDGE('',*,*,#15862,.F.);
#22324=ORIENTED_EDGE('',*,*,#15870,.T.);
#22325=ORIENTED_EDGE('',*,*,#15883,.F.);
#22326=ORIENTED_EDGE('',*,*,#15893,.F.);
#22327=ORIENTED_EDGE('',*,*,#15825,.F.);
#22328=ORIENTED_EDGE('',*,*,#15896,.T.);
#22329=ORIENTED_EDGE('',*,*,#15788,.T.);
#22330=ORIENTED_EDGE('',*,*,#15897,.T.);
#22331=ORIENTED_EDGE('',*,*,#15828,.F.);
#22332=ORIENTED_EDGE('',*,*,#15848,.T.);
#22333=ORIENTED_EDGE('',*,*,#15789,.T.);
#22334=ORIENTED_EDGE('',*,*,#15896,.F.);
#22335=ORIENTED_EDGE('',*,*,#15819,.F.);
#22336=ORIENTED_EDGE('',*,*,#15898,.T.);
#22337=ORIENTED_EDGE('',*,*,#15794,.T.);
#22338=ORIENTED_EDGE('',*,*,#15851,.F.);
#22339=ORIENTED_EDGE('',*,*,#15822,.F.);
#22340=ORIENTED_EDGE('',*,*,#15897,.F.);
#22341=ORIENTED_EDGE('',*,*,#15795,.T.);
#22342=ORIENTED_EDGE('',*,*,#15898,.F.);
#22343=ORIENTED_EDGE('',*,*,#15835,.F.);
#22344=ORIENTED_EDGE('',*,*,#15899,.F.);
#22345=ORIENTED_EDGE('',*,*,#15887,.F.);
#22346=ORIENTED_EDGE('',*,*,#15900,.T.);
#22347=ORIENTED_EDGE('',*,*,#15832,.F.);
#22348=ORIENTED_EDGE('',*,*,#15901,.F.);
#22349=ORIENTED_EDGE('',*,*,#15890,.F.);
#22350=ORIENTED_EDGE('',*,*,#15899,.T.);
#22351=ORIENTED_EDGE('',*,*,#15829,.F.);
#22352=ORIENTED_EDGE('',*,*,#15840,.F.);
#22353=ORIENTED_EDGE('',*,*,#15892,.F.);
#22354=ORIENTED_EDGE('',*,*,#15901,.T.);
#22355=ORIENTED_EDGE('',*,*,#15837,.F.);
#22356=ORIENTED_EDGE('',*,*,#15900,.F.);
#22357=ORIENTED_EDGE('',*,*,#15884,.F.);
#22358=ORIENTED_EDGE('',*,*,#15845,.T.);
#25072=CONICAL_SURFACE('',#28432,0.912322330470337,1.1780972450962);
#25073=CONICAL_SURFACE('',#28435,0.855,0.785398163397455);
#25074=CONICAL_SURFACE('',#28442,0.822677669529664,0.392699081698729);
#25075=CONICAL_SURFACE('',#28446,0.822677669529664,0.392699081698729);
#25076=CONICAL_SURFACE('',#28448,0.855,0.785398163397456);
#25077=CONICAL_SURFACE('',#28450,0.912322330470337,1.1780972450962);
#25078=CONICAL_SURFACE('',#28457,0.782322330470333,0.392699081698756);
#25079=CONICAL_SURFACE('',#28461,0.782322330470341,0.392699081698706);
#25080=CONICAL_SURFACE('',#28465,0.782322330470341,0.392699081698703);
#25081=CONICAL_SURFACE('',#28469,0.782322330470335,0.39269908169872);
#25082=CONICAL_SURFACE('',#28480,0.749999999999996,0.785398163397465);
#25083=CONICAL_SURFACE('',#28482,0.749999999999995,0.785398163397465);
#25084=CONICAL_SURFACE('',#28484,0.692677669529668,1.17809724509619);
#25085=CONICAL_SURFACE('',#28487,0.692677669529657,1.1780972450962);
#25086=CONICAL_SURFACE('',#28490,0.692677669529655,1.17809724509618);
#25087=CONICAL_SURFACE('',#28493,0.692677669529664,1.1780972450962);
#25088=CONICAL_SURFACE('',#28495,0.749999999999995,0.785398163397466);
#25089=CONICAL_SURFACE('',#28498,0.750000000000004,0.785398163397447);
#25090=CONICAL_SURFACE('',#28502,0.782322330470341,0.392699081698714);
#25091=CONICAL_SURFACE('',#28504,0.782322330470333,0.392699081698756);
#25092=CONICAL_SURFACE('',#28506,0.782322330470335,0.39269908169872);
#25093=CONICAL_SURFACE('',#28510,0.782322330470341,0.392699081698703);
#25094=CONICAL_SURFACE('',#28513,0.749999999999996,0.785398163397466);
#25095=CONICAL_SURFACE('',#28515,0.750000000000004,0.785398163397447);
#25096=CONICAL_SURFACE('',#28518,0.750000000000004,0.785398163397447);
#25097=CONICAL_SURFACE('',#28520,0.750000000000004,0.785398163397447);
#26100=ADVANCED_FACE('',(#3512),#25072,.F.);
#26101=ADVANCED_FACE('',(#3513),#25073,.F.);
#26102=ADVANCED_FACE('',(#3514,#1642),#2159,.T.);
#26103=ADVANCED_FACE('',(#3515),#25074,.F.);
#26104=ADVANCED_FACE('',(#3516),#1402,.F.);
#26105=ADVANCED_FACE('',(#3517),#25075,.F.);
#26106=ADVANCED_FACE('',(#3518),#25076,.F.);
#26107=ADVANCED_FACE('',(#3519),#25077,.F.);
#26108=ADVANCED_FACE('',(#3520,#1643),#2160,.F.);
#26109=ADVANCED_FACE('',(#3521),#25078,.T.);
#26110=ADVANCED_FACE('',(#3522),#2161,.T.);
#26111=ADVANCED_FACE('',(#3523),#25079,.T.);
#26112=ADVANCED_FACE('',(#3524),#2162,.T.);
#26113=ADVANCED_FACE('',(#3525),#25080,.T.);
#26114=ADVANCED_FACE('',(#3526),#2163,.T.);
#26115=ADVANCED_FACE('',(#3527),#25081,.T.);
#26116=ADVANCED_FACE('',(#3528),#2164,.T.);
#26117=ADVANCED_FACE('',(#3529),#2165,.T.);
#26118=ADVANCED_FACE('',(#3530),#1403,.T.);
#26119=ADVANCED_FACE('',(#3531),#2166,.T.);
#26120=ADVANCED_FACE('',(#3532),#1404,.T.);
#26121=ADVANCED_FACE('',(#3533),#2167,.T.);
#26122=ADVANCED_FACE('',(#3534),#25082,.T.);
#26123=ADVANCED_FACE('',(#3535),#2168,.T.);
#26124=ADVANCED_FACE('',(#3536),#25083,.T.);
#26125=ADVANCED_FACE('',(#3537),#2169,.T.);
#26126=ADVANCED_FACE('',(#3538),#25084,.T.);
#26127=ADVANCED_FACE('',(#3539),#2170,.T.);
#26128=ADVANCED_FACE('',(#3540),#25085,.T.);
#26129=ADVANCED_FACE('',(#3541),#2171,.T.);
#26130=ADVANCED_FACE('',(#3542),#25086,.T.);
#26131=ADVANCED_FACE('',(#3543),#2172,.T.);
#26132=ADVANCED_FACE('',(#3544),#25087,.T.);
#26133=ADVANCED_FACE('',(#3545),#25088,.T.);
#26134=ADVANCED_FACE('',(#3546),#2173,.T.);
#26135=ADVANCED_FACE('',(#3547),#25089,.T.);
#26136=ADVANCED_FACE('',(#3548),#2174,.T.);
#26137=ADVANCED_FACE('',(#3549),#2175,.T.);
#26138=ADVANCED_FACE('',(#3550),#25090,.T.);
#26139=ADVANCED_FACE('',(#3551),#2176,.T.);
#26140=ADVANCED_FACE('',(#3552),#25091,.T.);
#26141=ADVANCED_FACE('',(#3553),#2177,.T.);
#26142=ADVANCED_FACE('',(#3554),#25092,.T.);
#26143=ADVANCED_FACE('',(#3555),#2178,.T.);
#26144=ADVANCED_FACE('',(#3556),#25093,.T.);
#26145=ADVANCED_FACE('',(#3557),#25094,.T.);
#26146=ADVANCED_FACE('',(#3558),#2179,.T.);
#26147=ADVANCED_FACE('',(#3559),#25095,.T.);
#26148=ADVANCED_FACE('',(#3560),#2180,.T.);
#26149=ADVANCED_FACE('',(#3561),#2181,.T.);
#26150=ADVANCED_FACE('',(#3562),#25096,.T.);
#26151=ADVANCED_FACE('',(#3563),#2182,.T.);
#26152=ADVANCED_FACE('',(#3564),#25097,.T.);
#26153=ADVANCED_FACE('',(#3565),#1405,.T.);
#26154=ADVANCED_FACE('',(#3566),#2183,.T.);
#26155=ADVANCED_FACE('',(#3567),#1406,.T.);
#26156=ADVANCED_FACE('',(#3568),#2184,.T.);
#26679=CLOSED_SHELL('',(#26100,#26101,#26102,#26103,#26104,#26105,#26106,
#26107,#26108,#26109,#26110,#26111,#26112,#26113,#26114,#26115,#26116,#26117,
#26118,#26119,#26120,#26121,#26122,#26123,#26124,#26125,#26126,#26127,#26128,
#26129,#26130,#26131,#26132,#26133,#26134,#26135,#26136,#26137,#26138,#26139,
#26140,#26141,#26142,#26143,#26144,#26145,#26146,#26147,#26148,#26149,#26150,
#26151,#26152,#26153,#26154,#26155,#26156));
#28431=AXIS2_PLACEMENT_3D('',#63238,#33764,#33765);
#28432=AXIS2_PLACEMENT_3D('',#63239,#33766,#33767);
#28433=AXIS2_PLACEMENT_3D('',#63241,#33768,#33769);
#28434=AXIS2_PLACEMENT_3D('',#63244,#33771,#33772);
#28435=AXIS2_PLACEMENT_3D('',#63245,#33773,#33774);
#28436=AXIS2_PLACEMENT_3D('',#63248,#33776,#33777);
#28437=AXIS2_PLACEMENT_3D('',#63249,#33778,#33779);
#28438=AXIS2_PLACEMENT_3D('',#63254,#33781,#33782);
#28439=AXIS2_PLACEMENT_3D('',#63258,#33784,#33785);
#28440=AXIS2_PLACEMENT_3D('',#63262,#33787,#33788);
#28441=AXIS2_PLACEMENT_3D('',#63265,#33790,#33791);
#28442=AXIS2_PLACEMENT_3D('',#63266,#33792,#33793);
#28443=AXIS2_PLACEMENT_3D('',#63269,#33795,#33796);
#28444=AXIS2_PLACEMENT_3D('',#63270,#33797,#33798);
#28445=AXIS2_PLACEMENT_3D('',#63272,#33799,#33800);
#28446=AXIS2_PLACEMENT_3D('',#63274,#33802,#33803);
#28447=AXIS2_PLACEMENT_3D('',#63276,#33804,#33805);
#28448=AXIS2_PLACEMENT_3D('',#63278,#33807,#33808);
#28449=AXIS2_PLACEMENT_3D('',#63280,#33809,#33810);
#28450=AXIS2_PLACEMENT_3D('',#63282,#33812,#33813);
#28451=AXIS2_PLACEMENT_3D('',#63285,#33815,#33816);
#28452=AXIS2_PLACEMENT_3D('',#63286,#33817,#33818);
#28453=AXIS2_PLACEMENT_3D('',#63291,#33820,#33821);
#28454=AXIS2_PLACEMENT_3D('',#63295,#33823,#33824);
#28455=AXIS2_PLACEMENT_3D('',#63299,#33826,#33827);
#28456=AXIS2_PLACEMENT_3D('',#63302,#33829,#33830);
#28457=AXIS2_PLACEMENT_3D('',#63303,#33831,#33832);
#28458=AXIS2_PLACEMENT_3D('',#63308,#33834,#33835);
#28459=AXIS2_PLACEMENT_3D('',#63311,#33837,#33838);
#28460=AXIS2_PLACEMENT_3D('',#63312,#33839,#33840);
#28461=AXIS2_PLACEMENT_3D('',#63318,#33844,#33845);
#28462=AXIS2_PLACEMENT_3D('',#63322,#33847,#33848);
#28463=AXIS2_PLACEMENT_3D('',#63323,#33849,#33850);
#28464=AXIS2_PLACEMENT_3D('',#63324,#33851,#33852);
#28465=AXIS2_PLACEMENT_3D('',#63330,#33856,#33857);
#28466=AXIS2_PLACEMENT_3D('',#63334,#33859,#33860);
#28467=AXIS2_PLACEMENT_3D('',#63335,#33861,#33862);
#28468=AXIS2_PLACEMENT_3D('',#63336,#33863,#33864);
#28469=AXIS2_PLACEMENT_3D('',#63342,#33868,#33869);
#28470=AXIS2_PLACEMENT_3D('',#63346,#33871,#33872);
#28471=AXIS2_PLACEMENT_3D('',#63347,#33873,#33874);
#28472=AXIS2_PLACEMENT_3D('',#63348,#33875,#33876);
#28473=AXIS2_PLACEMENT_3D('',#63351,#33879,#33880);
#28474=AXIS2_PLACEMENT_3D('',#63357,#33884,#33885);
#28475=AXIS2_PLACEMENT_3D('',#63360,#33887,#33888);
#28476=AXIS2_PLACEMENT_3D('',#63361,#33889,#33890);
#28477=AXIS2_PLACEMENT_3D('',#63365,#33893,#33894);
#28478=AXIS2_PLACEMENT_3D('',#63368,#33896,#33897);
#28479=AXIS2_PLACEMENT_3D('',#63369,#33898,#33899);
#28480=AXIS2_PLACEMENT_3D('',#63372,#33902,#33903);
#28481=AXIS2_PLACEMENT_3D('',#63374,#33905,#33906);
#28482=AXIS2_PLACEMENT_3D('',#63376,#33908,#33909);
#28483=AXIS2_PLACEMENT_3D('',#63378,#33911,#33912);
#28484=AXIS2_PLACEMENT_3D('',#63384,#33916,#33917);
#28485=AXIS2_PLACEMENT_3D('',#63387,#33919,#33920);
#28486=AXIS2_PLACEMENT_3D('',#63388,#33921,#33922);
#28487=AXIS2_PLACEMENT_3D('',#63392,#33925,#33926);
#28488=AXIS2_PLACEMENT_3D('',#63395,#33928,#33929);
#28489=AXIS2_PLACEMENT_3D('',#63396,#33930,#33931);
#28490=AXIS2_PLACEMENT_3D('',#63400,#33934,#33935);
#28491=AXIS2_PLACEMENT_3D('',#63403,#33937,#33938);
#28492=AXIS2_PLACEMENT_3D('',#63404,#33939,#33940);
#28493=AXIS2_PLACEMENT_3D('',#63408,#33943,#33944);
#28494=AXIS2_PLACEMENT_3D('',#63409,#33945,#33946);
#28495=AXIS2_PLACEMENT_3D('',#63410,#33947,#33948);
#28496=AXIS2_PLACEMENT_3D('',#63414,#33950,#33951);
#28497=AXIS2_PLACEMENT_3D('',#63416,#33953,#33954);
#28498=AXIS2_PLACEMENT_3D('',#63420,#33957,#33958);
#28499=AXIS2_PLACEMENT_3D('',#63423,#33960,#33961);
#28500=AXIS2_PLACEMENT_3D('',#63424,#33962,#33963);
#28501=AXIS2_PLACEMENT_3D('',#63428,#33966,#33967);
#28502=AXIS2_PLACEMENT_3D('',#63431,#33970,#33971);
#28503=AXIS2_PLACEMENT_3D('',#63433,#33973,#33974);
#28504=AXIS2_PLACEMENT_3D('',#63435,#33976,#33977);
#28505=AXIS2_PLACEMENT_3D('',#63437,#33979,#33980);
#28506=AXIS2_PLACEMENT_3D('',#63443,#33984,#33985);
#28507=AXIS2_PLACEMENT_3D('',#63447,#33987,#33988);
#28508=AXIS2_PLACEMENT_3D('',#63448,#33989,#33990);
#28509=AXIS2_PLACEMENT_3D('',#63449,#33991,#33992);
#28510=AXIS2_PLACEMENT_3D('',#63455,#33996,#33997);
#28511=AXIS2_PLACEMENT_3D('',#63456,#33998,#33999);
#28512=AXIS2_PLACEMENT_3D('',#63457,#34000,#34001);
#28513=AXIS2_PLACEMENT_3D('',#63458,#34002,#34003);
#28514=AXIS2_PLACEMENT_3D('',#63461,#34006,#34007);
#28515=AXIS2_PLACEMENT_3D('',#63463,#34009,#34010);
#28516=AXIS2_PLACEMENT_3D('',#63464,#34011,#34012);
#28517=AXIS2_PLACEMENT_3D('',#63465,#34013,#34014);
#28518=AXIS2_PLACEMENT_3D('',#63468,#34017,#34018);
#28519=AXIS2_PLACEMENT_3D('',#63469,#34019,#34020);
#28520=AXIS2_PLACEMENT_3D('',#63471,#34022,#34023);
#28521=AXIS2_PLACEMENT_3D('',#63472,#34024,#34025);
#28522=AXIS2_PLACEMENT_3D('',#63475,#34028,#34029);
#28523=AXIS2_PLACEMENT_3D('',#63477,#34031,#34032);
#28524=AXIS2_PLACEMENT_3D('',#63478,#34033,#34034);
#33764=DIRECTION('axis',(0.,0.,1.));
#33765=DIRECTION('refdir',(1.,0.,0.));
#33766=DIRECTION('center_axis',(0.,1.50614812182896E-15,1.));
#33767=DIRECTION('ref_axis',(1.,2.918397135658E-17,0.));
#33768=DIRECTION('center_axis',(0.,0.,-1.));
#33769=DIRECTION('ref_axis',(1.,6.12323399573679E-17,0.));
#33770=DIRECTION('',(-0.923879532511297,6.62558070326733E-16,0.382683432365065));
#33771=DIRECTION('center_axis',(0.,0.,1.));
#33772=DIRECTION('ref_axis',(1.,0.,0.));
#33773=DIRECTION('center_axis',(0.,0.,1.));
#33774=DIRECTION('ref_axis',(1.,0.,0.));
#33775=DIRECTION('',(0.707106781186552,8.65956056235499E-17,-0.707106781186543));
#33776=DIRECTION('center_axis',(1.617924002207E-32,-2.64227041353223E-16,
1.));
#33777=DIRECTION('ref_axis',(1.,6.12323399573677E-17,0.));
#33778=DIRECTION('center_axis',(0.,0.,1.));
#33779=DIRECTION('ref_axis',(1.,0.,0.));
#33780=DIRECTION('',(0.,1.,0.));
#33781=DIRECTION('center_axis',(0.,0.,-1.));
#33782=DIRECTION('ref_axis',(-1.,-6.6613381477509E-15,0.));
#33783=DIRECTION('',(-1.,0.,0.));
#33784=DIRECTION('center_axis',(0.,0.,-1.));
#33785=DIRECTION('ref_axis',(0.,-1.,0.));
#33786=DIRECTION('',(0.,-1.,0.));
#33787=DIRECTION('center_axis',(0.,0.,-1.));
#33788=DIRECTION('ref_axis',(1.,-2.22044604925032E-15,0.));
#33789=DIRECTION('',(1.,0.,0.));
#33790=DIRECTION('center_axis',(0.,0.,-1.));
#33791=DIRECTION('ref_axis',(-4.4408920985006E-15,1.,0.));
#33792=DIRECTION('center_axis',(0.,-6.02855361754257E-16,1.));
#33793=DIRECTION('ref_axis',(1.,3.12740491884801E-17,0.));
#33794=DIRECTION('',(0.382683432365095,6.1579899433011E-16,-0.923879532511285));
#33795=DIRECTION('center_axis',(0.,0.,-1.));
#33796=DIRECTION('ref_axis',(1.,0.,0.));
#33797=DIRECTION('center_axis',(0.,0.,1.));
#33798=DIRECTION('ref_axis',(1.,0.,0.));
#33799=DIRECTION('center_axis',(0.,0.,1.));
#33800=DIRECTION('ref_axis',(1.,0.,0.));
#33801=DIRECTION('',(0.,0.,1.));
#33802=DIRECTION('center_axis',(0.,6.02855361754257E-16,-1.));
#33803=DIRECTION('ref_axis',(1.,-3.12740491884801E-17,0.));
#33804=DIRECTION('center_axis',(2.4268860033105E-32,3.96340562029835E-16,
-1.));
#33805=DIRECTION('ref_axis',(1.,-6.12323399573677E-17,0.));
#33806=DIRECTION('',(0.382683432365094,-6.1579899433011E-16,0.923879532511285));
#33807=DIRECTION('center_axis',(0.,0.,-1.));
#33808=DIRECTION('ref_axis',(1.,0.,0.));
#33809=DIRECTION('center_axis',(3.90858224776604E-33,6.38319922199173E-17,
1.));
#33810=DIRECTION('ref_axis',(1.,-6.12323399573679E-17,0.));
#33811=DIRECTION('',(0.707106781186553,-8.659560562355E-17,0.707106781186542));
#33812=DIRECTION('center_axis',(0.,-1.50614812182896E-15,-1.));
#33813=DIRECTION('ref_axis',(1.,-2.918397135658E-17,0.));
#33814=DIRECTION('',(-0.923879532511297,-6.62558070326733E-16,-0.382683432365064));
#33815=DIRECTION('center_axis',(0.,0.,-1.));
#33816=DIRECTION('ref_axis',(1.,0.,0.));
#33817=DIRECTION('center_axis',(0.,0.,1.));
#33818=DIRECTION('ref_axis',(1.,0.,0.));
#33819=DIRECTION('',(0.,-1.,0.));
#33820=DIRECTION('center_axis',(0.,0.,1.));
#33821=DIRECTION('ref_axis',(-4.4408920985006E-15,1.,0.));
#33822=DIRECTION('',(-1.,0.,0.));
#33823=DIRECTION('center_axis',(0.,0.,1.));
#33824=DIRECTION('ref_axis',(1.,-2.22044604925032E-15,0.));
#33825=DIRECTION('',(0.,1.,0.));
#33826=DIRECTION('center_axis',(0.,0.,1.));
#33827=DIRECTION('ref_axis',(0.,-1.,0.));
#33828=DIRECTION('',(1.,0.,0.));
#33829=DIRECTION('center_axis',(0.,0.,1.));
#33830=DIRECTION('ref_axis',(-1.,-6.6613381477509E-15,0.));
#33831=DIRECTION('center_axis',(0.,0.,-1.));
#33832=DIRECTION('ref_axis',(1.,-2.27062013982434E-15,0.));
#33833=DIRECTION('',(0.,-0.382683432365106,0.92387953251128));
#33834=DIRECTION('center_axis',(4.72225197640989E-30,2.03272489022952E-15,
-1.));
#33835=DIRECTION('ref_axis',(1.,-2.32311416026233E-15,0.));
#33836=DIRECTION('',(0.382683432365098,-9.61357393951414E-15,-0.923879532511283));
#33837=DIRECTION('center_axis',(0.,0.,1.));
#33838=DIRECTION('ref_axis',(1.,-2.22044604925032E-15,0.));
#33839=DIRECTION('center_axis',(0.,0.923879532511288,0.382683432365087));
#33840=DIRECTION('ref_axis',(0.,-0.382683432365087,0.923879532511288));
#33841=DIRECTION('',(0.,-0.382683432365087,0.923879532511288));
#33842=DIRECTION('',(1.,0.,0.));
#33843=DIRECTION('',(-1.,0.,0.));
#33844=DIRECTION('center_axis',(0.,0.,-1.));
#33845=DIRECTION('ref_axis',(-4.54124027964863E-15,1.,0.));
#33846=DIRECTION('',(0.382683432365071,0.,0.923879532511295));
#33847=DIRECTION('center_axis',(-5.80778540065573E-16,-2.69842970080559E-30,
-1.));
#33848=DIRECTION('ref_axis',(-4.64622832052459E-15,1.,0.));
#33849=DIRECTION('center_axis',(0.,0.,1.));
#33850=DIRECTION('ref_axis',(-4.4408920985006E-15,1.,0.));
#33851=DIRECTION('center_axis',(-0.923879532511282,0.,0.382683432365102));
#33852=DIRECTION('ref_axis',(0.382683432365102,0.,0.923879532511282));
#33853=DIRECTION('',(0.382683432365101,0.,0.923879532511282));
#33854=DIRECTION('',(0.,1.,0.));
#33855=DIRECTION('',(0.,-1.,0.));
#33856=DIRECTION('center_axis',(0.,0.,-1.));
#33857=DIRECTION('ref_axis',(-1.,-6.81186041947294E-15,0.));
#33858=DIRECTION('',(0.,0.382683432365072,0.923879532511294));
#33859=DIRECTION('center_axis',(-4.04764455120838E-30,5.80778540065573E-16,
-1.));
#33860=DIRECTION('ref_axis',(-1.,-6.96934248078688E-15,0.));
#33861=DIRECTION('center_axis',(0.,0.,1.));
#33862=DIRECTION('ref_axis',(-1.,-6.6613381477509E-15,0.));
#33863=DIRECTION('center_axis',(0.,-0.923879532511288,0.382683432365087));
#33864=DIRECTION('ref_axis',(0.,-0.382683432365087,-0.923879532511288));
#33865=DIRECTION('',(0.,0.382683432365087,0.923879532511288));
#33866=DIRECTION('',(-1.,0.,0.));
#33867=DIRECTION('',(1.,0.,0.));
#33868=DIRECTION('center_axis',(0.,0.,-1.));
#33869=DIRECTION('ref_axis',(0.,-1.,0.));
#33870=DIRECTION('',(-0.382683432365058,0.,0.9238795325113));
#33871=DIRECTION('center_axis',(-2.61350343029512E-15,0.,-1.));
#33872=DIRECTION('ref_axis',(0.,-1.,0.));
#33873=DIRECTION('center_axis',(0.,0.,1.));
#33874=DIRECTION('ref_axis',(0.,-1.,0.));
#33875=DIRECTION('center_axis',(0.923879532511282,0.,0.382683432365101));
#33876=DIRECTION('ref_axis',(0.382683432365101,0.,-0.923879532511282));
#33877=DIRECTION('',(0.,-1.,0.));
#33878=DIRECTION('',(0.,1.,0.));
#33879=DIRECTION('center_axis',(-1.,0.,0.));
#33880=DIRECTION('ref_axis',(0.,-1.,0.));
#33881=DIRECTION('',(0.,0.,1.));
#33882=DIRECTION('',(0.,1.,0.));
#33883=DIRECTION('',(0.,0.,1.));
#33884=DIRECTION('center_axis',(0.,0.,1.));
#33885=DIRECTION('ref_axis',(-4.4408920985006E-15,1.,0.));
#33886=DIRECTION('',(0.,0.,1.));
#33887=DIRECTION('center_axis',(0.,0.,-1.));
#33888=DIRECTION('ref_axis',(-4.4408920985006E-15,1.,0.));
#33889=DIRECTION('center_axis',(0.,1.,0.));
#33890=DIRECTION('ref_axis',(-1.,0.,0.));
#33891=DIRECTION('',(0.,0.,1.));
#33892=DIRECTION('',(1.,0.,0.));
#33893=DIRECTION('center_axis',(0.,0.,1.));
#33894=DIRECTION('ref_axis',(1.,-2.22044604925032E-15,0.));
#33895=DIRECTION('',(0.,0.,1.));
#33896=DIRECTION('center_axis',(0.,0.,-1.));
#33897=DIRECTION('ref_axis',(1.,-2.22044604925032E-15,0.));
#33898=DIRECTION('center_axis',(0.,-0.707106781186549,0.707106781186546));
#33899=DIRECTION('ref_axis',(1.,0.,0.));
#33900=DIRECTION('',(0.,0.707106781186546,0.707106781186549));
#33901=DIRECTION('',(0.,0.707106781186546,0.707106781186549));
#33902=DIRECTION('center_axis',(0.,0.,-1.));
#33903=DIRECTION('ref_axis',(0.,-1.,0.));
#33904=DIRECTION('',(-0.707106781186552,0.,0.707106781186543));
#33905=DIRECTION('center_axis',(0.707106781186543,0.,0.707106781186552));
#33906=DIRECTION('ref_axis',(0.707106781186552,0.,-0.707106781186543));
#33907=DIRECTION('',(-0.707106781186552,6.28036983473505E-15,0.707106781186543));
#33908=DIRECTION('center_axis',(0.,0.,-1.));
#33909=DIRECTION('ref_axis',(1.,-2.22044604925032E-15,0.));
#33910=DIRECTION('',(0.,-0.707106781186562,0.707106781186533));
#33911=DIRECTION('center_axis',(-0.382683432365119,0.,-0.923879532511275));
#33912=DIRECTION('ref_axis',(-0.923879532511275,0.,0.382683432365119));
#33913=DIRECTION('',(-0.923879532511278,9.61357393951443E-15,0.382683432365112));
#33914=DIRECTION('',(0.,1.,0.));
#33915=DIRECTION('',(0.923879532511278,0.,-0.382683432365112));
#33916=DIRECTION('center_axis',(0.,0.,1.));
#33917=DIRECTION('ref_axis',(-1.,-6.97217532708781E-15,0.));
#33918=DIRECTION('',(0.,-0.923879532511291,0.38268343236508));
#33919=DIRECTION('center_axis',(-5.47062821941541E-31,7.54888803857301E-17,
-1.));
#33920=DIRECTION('ref_axis',(-1.,-7.24693251703008E-15,0.));
#33921=DIRECTION('center_axis',(0.,-0.382683432365091,-0.923879532511286));
#33922=DIRECTION('ref_axis',(-1.,0.,0.));
#33923=DIRECTION('',(0.,-0.923879532511286,0.382683432365091));
#33924=DIRECTION('',(-1.,0.,0.));
#33925=DIRECTION('center_axis',(0.,0.,1.));
#33926=DIRECTION('ref_axis',(0.,-1.,0.));
#33927=DIRECTION('',(0.923879532511292,0.,0.382683432365078));
#33928=DIRECTION('center_axis',(1.4342887273289E-15,0.,-1.));
#33929=DIRECTION('ref_axis',(0.,-1.,0.));
#33930=DIRECTION('center_axis',(0.382683432365081,0.,-0.92387953251129));
#33931=DIRECTION('ref_axis',(-0.92387953251129,0.,-0.382683432365081));
#33932=DIRECTION('',(0.92387953251129,-9.61357393951456E-15,0.382683432365082));
#33933=DIRECTION('',(0.,-1.,0.));
#33934=DIRECTION('center_axis',(0.,0.,1.));
#33935=DIRECTION('ref_axis',(1.,-2.32405844236264E-15,0.));
#33936=DIRECTION('',(0.,0.923879532511303,0.382683432365051));
#33937=DIRECTION('center_axis',(-3.28237693164936E-30,-1.35879984694316E-15,
-1.));
#33938=DIRECTION('ref_axis',(1.,-2.41564417234341E-15,0.));
#33939=DIRECTION('center_axis',(0.,0.382683432365091,-0.923879532511286));
#33940=DIRECTION('ref_axis',(-1.,0.,0.));
#33941=DIRECTION('',(0.,0.923879532511286,0.382683432365091));
#33942=DIRECTION('',(1.,0.,0.));
#33943=DIRECTION('center_axis',(0.,0.,1.));
#33944=DIRECTION('ref_axis',(-4.64811688472521E-15,1.,0.));
#33945=DIRECTION('center_axis',(-6.79399923471573E-16,-3.28237693164927E-30,
-1.));
#33946=DIRECTION('ref_axis',(-4.83128834468673E-15,1.,0.));
#33947=DIRECTION('center_axis',(0.,0.,1.));
#33948=DIRECTION('ref_axis',(1.,-2.22044604925032E-15,0.));
#33949=DIRECTION('',(0.,0.707106781186562,0.707106781186533));
#33950=DIRECTION('center_axis',(-4.55360012010954E-30,-1.96012757272133E-15,
1.));
#33951=DIRECTION('ref_axis',(1.,-2.32311416026233E-15,0.));
#33952=DIRECTION('',(0.707106781186578,-6.28036983473483E-15,0.707106781186517));
#33953=DIRECTION('center_axis',(0.,0.707106781186549,-0.707106781186546));
#33954=DIRECTION('ref_axis',(-1.,0.,0.));
#33955=DIRECTION('',(0.,0.707106781186546,0.707106781186549));
#33956=DIRECTION('',(-1.,0.,0.));
#33957=DIRECTION('center_axis',(0.,0.,1.));
#33958=DIRECTION('ref_axis',(-4.4408920985006E-15,1.,0.));
#33959=DIRECTION('',(0.707106781186552,0.,-0.707106781186543));
#33960=DIRECTION('center_axis',(-1.81493293770492E-15,-8.43259281501748E-30,
1.));
#33961=DIRECTION('ref_axis',(-4.64622832052459E-15,1.,0.));
#33962=DIRECTION('center_axis',(-0.707106781186543,0.,-0.707106781186552));
#33963=DIRECTION('ref_axis',(-0.707106781186552,0.,0.707106781186543));
#33964=DIRECTION('',(-0.707106781186552,6.28036983473505E-15,0.707106781186543));
#33965=DIRECTION('',(0.,-1.,0.));
#33966=DIRECTION('center_axis',(-0.923879532511297,0.,-0.382683432365065));
#33967=DIRECTION('ref_axis',(-0.382683432365065,0.,0.923879532511297));
#33968=DIRECTION('',(0.382683432365068,0.,-0.923879532511296));
#33969=DIRECTION('',(-0.382683432365068,0.,0.923879532511296));
#33970=DIRECTION('center_axis',(0.,0.,1.));
#33971=DIRECTION('ref_axis',(-4.54124027964863E-15,1.,0.));
#33972=DIRECTION('',(0.,-0.382683432365081,-0.923879532511291));
#33973=DIRECTION('center_axis',(0.,0.923879532511287,-0.382683432365088));
#33974=DIRECTION('ref_axis',(0.,0.382683432365088,0.923879532511287));
#33975=DIRECTION('',(0.,-0.3826834323651,-0.923879532511283));
#33976=DIRECTION('center_axis',(0.,0.,1.));
#33977=DIRECTION('ref_axis',(1.,-2.27062013982434E-15,0.));
#33978=DIRECTION('',(-0.382683432365108,9.6135739395144E-15,-0.923879532511279));
#33979=DIRECTION('center_axis',(0.92387953251128,0.,-0.382683432365108));
#33980=DIRECTION('ref_axis',(-0.382683432365108,0.,-0.92387953251128));
#33981=DIRECTION('',(-0.382683432365102,0.,-0.923879532511282));
#33982=DIRECTION('',(0.,1.,0.));
#33983=DIRECTION('',(0.,-1.,0.));
#33984=DIRECTION('center_axis',(0.,0.,1.));
#33985=DIRECTION('ref_axis',(0.,-1.,0.));
#33986=DIRECTION('',(0.,0.382683432365081,-0.923879532511291));
#33987=DIRECTION('center_axis',(2.68610074780331E-15,0.,1.));
#33988=DIRECTION('ref_axis',(0.,-1.,0.));
#33989=DIRECTION('center_axis',(0.,0.,-1.));
#33990=DIRECTION('ref_axis',(0.,-1.,0.));
#33991=DIRECTION('center_axis',(0.,-0.923879532511287,-0.382683432365088));
#33992=DIRECTION('ref_axis',(0.,0.382683432365088,-0.923879532511287));
#33993=DIRECTION('',(0.,0.38268343236509,-0.923879532511287));
#33994=DIRECTION('',(1.,0.,0.));
#33995=DIRECTION('',(-1.,0.,0.));
#33996=DIRECTION('center_axis',(0.,0.,1.));
#33997=DIRECTION('ref_axis',(-1.,-6.81186041947294E-15,0.));
#33998=DIRECTION('center_axis',(3.54168898230734E-30,-5.08181222557377E-16,
1.));
#33999=DIRECTION('ref_axis',(-1.,-6.96934248078688E-15,0.));
#34000=DIRECTION('center_axis',(0.,0.,-1.));
#34001=DIRECTION('ref_axis',(-1.,-6.6613381477509E-15,0.));
#34002=DIRECTION('center_axis',(0.,0.,1.));
#34003=DIRECTION('ref_axis',(0.,-1.,0.));
#34004=DIRECTION('',(0.707106781186552,0.,0.707106781186543));
#34005=DIRECTION('',(0.,-0.707106781186546,0.707106781186549));
#34006=DIRECTION('center_axis',(0.,-0.707106781186549,-0.707106781186546));
#34007=DIRECTION('ref_axis',(-1.,0.,0.));
#34008=DIRECTION('',(0.,-0.707106781186546,0.707106781186549));
#34009=DIRECTION('center_axis',(0.,0.,1.));
#34010=DIRECTION('ref_axis',(-1.,-6.66133814775091E-15,0.));
#34011=DIRECTION('center_axis',(0.707106781186517,0.,-0.707106781186578));
#34012=DIRECTION('ref_axis',(-0.707106781186578,0.,-0.707106781186517));
#34013=DIRECTION('center_axis',(-0.707106781186543,0.,0.707106781186552));
#34014=DIRECTION('ref_axis',(0.707106781186552,0.,0.707106781186543));
#34015=DIRECTION('',(0.707106781186552,-6.28036983473505E-15,0.707106781186543));
#34016=DIRECTION('',(-0.707106781186552,0.,-0.707106781186543));
#34017=DIRECTION('center_axis',(0.,0.,-1.));
#34018=DIRECTION('ref_axis',(-1.,-6.66133814775091E-15,0.));
#34019=DIRECTION('center_axis',(0.,0.707106781186549,0.707106781186546));
#34020=DIRECTION('ref_axis',(1.,0.,0.));
#34021=DIRECTION('',(0.,-0.707106781186546,0.707106781186549));
#34022=DIRECTION('center_axis',(0.,0.,-1.));
#34023=DIRECTION('ref_axis',(-4.4408920985006E-15,1.,0.));
#34024=DIRECTION('center_axis',(0.,0.,1.));
#34025=DIRECTION('ref_axis',(0.,-1.,0.));
#34026=DIRECTION('',(0.,0.,1.));
#34027=DIRECTION('',(0.,0.,1.));
#34028=DIRECTION('center_axis',(0.,-1.,0.));
#34029=DIRECTION('ref_axis',(1.,0.,0.));
#34030=DIRECTION('',(0.,0.,1.));
#34031=DIRECTION('center_axis',(0.,0.,1.));
#34032=DIRECTION('ref_axis',(-1.,-6.6613381477509E-15,0.));
#34033=DIRECTION('center_axis',(1.,0.,0.));
#34034=DIRECTION('ref_axis',(0.,1.,0.));
#63238=CARTESIAN_POINT('',(0.,0.,0.));
#63239=CARTESIAN_POINT('Origin',(33.6,-2.66251887604146E-17,1.78232233047034));
#63240=CARTESIAN_POINT('',(32.7303553390593,-3.94430452610506E-31,1.76464466094067));
#63241=CARTESIAN_POINT('Origin',(33.6,-5.32503775208292E-17,1.76464466094067));
#63242=CARTESIAN_POINT('',(32.645,-1.16953769318572E-16,1.8));
#63243=CARTESIAN_POINT('',(32.6876776695297,5.8476884659286E-17,1.78232233047034));
#63244=CARTESIAN_POINT('Origin',(33.6,0.,1.8));
#63245=CARTESIAN_POINT('Origin',(33.6,0.,1.75));
#63246=CARTESIAN_POINT('',(32.7596446609407,-2.05827695225079E-16,1.73535533905933));
#63247=CARTESIAN_POINT('',(32.745,-1.04707301327099E-16,1.75));
#63248=CARTESIAN_POINT('Origin',(33.6,-5.14569238062698E-17,1.73535533905933));
#63249=CARTESIAN_POINT('Origin',(33.6,0.,1.8));
#63250=CARTESIAN_POINT('',(30.5,-5.4,1.8));
#63251=CARTESIAN_POINT('',(30.5,5.4,1.8));
#63252=CARTESIAN_POINT('',(30.5,2.7,1.8));
#63253=CARTESIAN_POINT('',(31.2,-6.1,1.8));
#63254=CARTESIAN_POINT('Origin',(31.2,-5.4,1.8));
#63255=CARTESIAN_POINT('',(36.,-6.1,1.8));
#63256=CARTESIAN_POINT('',(32.4,-6.1,1.8));
#63257=CARTESIAN_POINT('',(36.7,-5.4,1.8));
#63258=CARTESIAN_POINT('Origin',(36.,-5.4,1.8));
#63259=CARTESIAN_POINT('',(36.7,5.4,1.8));
#63260=CARTESIAN_POINT('',(36.7,-2.7,1.8));
#63261=CARTESIAN_POINT('',(36.,6.1,1.8));
#63262=CARTESIAN_POINT('Origin',(36.,5.4,1.8));
#63263=CARTESIAN_POINT('',(31.2,6.1,1.8));
#63264=CARTESIAN_POINT('',(34.8,6.1,1.8));
#63265=CARTESIAN_POINT('Origin',(31.2,5.4,1.8));
#63266=CARTESIAN_POINT('Origin',(33.6,-2.57284619031349E-17,1.69267766952966));
#63267=CARTESIAN_POINT('',(32.795,9.85840673313619E-17,1.65));
#63268=CARTESIAN_POINT('',(32.7773223304703,-1.52205881278221E-16,1.69267766952966));
#63269=CARTESIAN_POINT('Origin',(33.6,0.,1.65));
#63270=CARTESIAN_POINT('Origin',(33.6,0.,0.99));
#63271=CARTESIAN_POINT('',(32.795,-9.85840673313619E-17,0.350000000000001));
#63272=CARTESIAN_POINT('Origin',(33.6,0.,0.350000000000001));
#63273=CARTESIAN_POINT('',(32.795,-9.85840673313619E-17,0.99));
#63274=CARTESIAN_POINT('Origin',(33.6,2.57284619031349E-17,0.307322330470336));
#63275=CARTESIAN_POINT('',(32.7596446609407,2.05827695225079E-16,0.264644660940671));
#63276=CARTESIAN_POINT('Origin',(33.6,5.14569238062698E-17,0.264644660940671));
#63277=CARTESIAN_POINT('',(32.7773223304703,1.52205881278221E-16,0.307322330470336));
#63278=CARTESIAN_POINT('Origin',(33.6,0.,0.25));
#63279=CARTESIAN_POINT('',(32.7303553390593,3.82104500966428E-31,0.235355339059325));
#63280=CARTESIAN_POINT('Origin',(33.6,5.32503775208292E-17,0.235355339059325));
#63281=CARTESIAN_POINT('',(32.745,1.04707301327099E-16,0.25));
#63282=CARTESIAN_POINT('Origin',(33.6,2.66251887604146E-17,0.217677669529663));
#63283=CARTESIAN_POINT('',(32.645,1.16953769318572E-16,0.2));
#63284=CARTESIAN_POINT('',(32.6876776695297,-5.8476884659286E-17,0.217677669529663));
#63285=CARTESIAN_POINT('Origin',(33.6,0.,0.2));
#63286=CARTESIAN_POINT('Origin',(33.6,0.,0.2));
#63287=CARTESIAN_POINT('',(30.55,5.4,0.2));
#63288=CARTESIAN_POINT('',(30.55,-5.4,0.2));
#63289=CARTESIAN_POINT('',(30.55,1.35,0.2));
#63290=CARTESIAN_POINT('',(31.2,6.05,0.2));
#63291=CARTESIAN_POINT('Origin',(31.2,5.4,0.2));
#63292=CARTESIAN_POINT('',(36.,6.04999999999999,0.2));
#63293=CARTESIAN_POINT('',(34.2,6.05,0.2));
#63294=CARTESIAN_POINT('',(36.65,5.4,0.2));
#63295=CARTESIAN_POINT('Origin',(36.,5.4,0.2));
#63296=CARTESIAN_POINT('',(36.65,-5.4,0.2));
#63297=CARTESIAN_POINT('',(36.65,-1.35,0.2));
#63298=CARTESIAN_POINT('',(36.,-6.05,0.2));
#63299=CARTESIAN_POINT('Origin',(36.,-5.4,0.2));
#63300=CARTESIAN_POINT('',(31.2,-6.05,0.2));
#63301=CARTESIAN_POINT('',(33.,-6.05,0.2));
#63302=CARTESIAN_POINT('Origin',(31.2,-5.4,0.2));
#63303=CARTESIAN_POINT('Origin',(36.,5.4,1.69267766952966));
#63304=CARTESIAN_POINT('',(36.,6.2,1.65));
#63305=CARTESIAN_POINT('',(36.,6.16464466094067,1.73535533905933));
#63306=CARTESIAN_POINT('',(36.,6.2,1.65));
#63307=CARTESIAN_POINT('',(36.7646446609407,5.4,1.73535533905933));
#63308=CARTESIAN_POINT('Origin',(36.,5.4,1.73535533905932));
#63309=CARTESIAN_POINT('',(36.8,5.4,1.65));
#63310=CARTESIAN_POINT('',(36.7646446609407,5.4,1.73535533905933));
#63311=CARTESIAN_POINT('Origin',(36.,5.4,1.65));
#63312=CARTESIAN_POINT('Origin',(35.4,6.18232233047034,1.69267766952966));
#63313=CARTESIAN_POINT('',(31.2,6.2,1.65));
#63314=CARTESIAN_POINT('',(31.2,6.16464466094067,1.73535533905933));
#63315=CARTESIAN_POINT('',(31.2,6.2,1.65));
#63316=CARTESIAN_POINT('',(35.4,6.16464466094067,1.73535533905933));
#63317=CARTESIAN_POINT('',(35.4,6.2,1.65));
#63318=CARTESIAN_POINT('Origin',(31.2,5.4,1.69267766952966));
#63319=CARTESIAN_POINT('',(30.4,5.4,1.65));
#63320=CARTESIAN_POINT('',(30.4353553390593,5.4,1.73535533905933));
#63321=CARTESIAN_POINT('',(30.4,5.4,1.65));
#63322=CARTESIAN_POINT('Origin',(31.2,5.4,1.73535533905933));
#63323=CARTESIAN_POINT('Origin',(31.2,5.4,1.65));
#63324=CARTESIAN_POINT('Origin',(30.4176776695297,4.05,1.69267766952966));
#63325=CARTESIAN_POINT('',(30.4,-5.4,1.65));
#63326=CARTESIAN_POINT('',(30.4353553390593,-5.4,1.73535533905933));
#63327=CARTESIAN_POINT('',(30.4,-5.4,1.65));
#63328=CARTESIAN_POINT('',(30.4353553390593,4.05,1.73535533905933));
#63329=CARTESIAN_POINT('',(30.4,4.05,1.65));
#63330=CARTESIAN_POINT('Origin',(31.2,-5.4,1.69267766952966));
#63331=CARTESIAN_POINT('',(31.2,-6.2,1.65));
#63332=CARTESIAN_POINT('',(31.2,-6.16464466094067,1.73535533905933));
#63333=CARTESIAN_POINT('',(31.2,-6.2,1.65));
#63334=CARTESIAN_POINT('Origin',(31.2,-5.4,1.73535533905933));
#63335=CARTESIAN_POINT('Origin',(31.2,-5.4,1.65));
#63336=CARTESIAN_POINT('Origin',(31.8,-6.18232233047034,1.69267766952966));
#63337=CARTESIAN_POINT('',(36.,-6.2,1.65));
#63338=CARTESIAN_POINT('',(36.,-6.16464466094067,1.73535533905933));
#63339=CARTESIAN_POINT('',(36.,-6.2,1.65));
#63340=CARTESIAN_POINT('',(31.8,-6.16464466094067,1.73535533905933));
#63341=CARTESIAN_POINT('',(31.8,-6.2,1.65));
#63342=CARTESIAN_POINT('Origin',(36.,-5.4,1.69267766952966));
#63343=CARTESIAN_POINT('',(36.8,-5.4,1.65));
#63344=CARTESIAN_POINT('',(36.7646446609407,-5.4,1.73535533905932));
#63345=CARTESIAN_POINT('',(36.8,-5.4,1.65));
#63346=CARTESIAN_POINT('Origin',(36.,-5.4,1.73535533905932));
#63347=CARTESIAN_POINT('Origin',(36.,-5.4,1.65));
#63348=CARTESIAN_POINT('Origin',(36.7823223304703,-4.05,1.69267766952967));
#63349=CARTESIAN_POINT('',(36.7646446609407,-4.05,1.73535533905933));
#63350=CARTESIAN_POINT('',(36.8,-4.05,1.65));
#63351=CARTESIAN_POINT('Origin',(30.4,5.4,0.2));
#63352=CARTESIAN_POINT('',(30.4,5.4,0.350000000000003));
#63353=CARTESIAN_POINT('',(30.4,5.4,0.2));
#63354=CARTESIAN_POINT('',(30.4,-5.4,0.350000000000003));
#63355=CARTESIAN_POINT('',(30.4,4.05,0.350000000000003));
#63356=CARTESIAN_POINT('',(30.4,-5.4,0.2));
#63357=CARTESIAN_POINT('Origin',(31.2,5.4,0.2));
#63358=CARTESIAN_POINT('',(31.2,6.2,0.350000000000001));
#63359=CARTESIAN_POINT('',(31.2,6.2,0.2));
#63360=CARTESIAN_POINT('Origin',(31.2,5.4,0.350000000000001));
#63361=CARTESIAN_POINT('Origin',(36.,6.2,0.2));
#63362=CARTESIAN_POINT('',(36.,6.2,0.35));
#63363=CARTESIAN_POINT('',(36.,6.2,0.2));
#63364=CARTESIAN_POINT('',(35.4,6.2,0.35));
#63365=CARTESIAN_POINT('Origin',(36.,5.4,0.2));
#63366=CARTESIAN_POINT('',(36.8,5.4,0.350000000000001));
#63367=CARTESIAN_POINT('',(36.8,5.4,0.2));
#63368=CARTESIAN_POINT('Origin',(36.,5.4,0.350000000000001));
#63369=CARTESIAN_POINT('Origin',(32.4,-6.15,1.75));
#63370=CARTESIAN_POINT('',(36.,-6.2,1.7));
#63371=CARTESIAN_POINT('',(31.2,-6.2,1.7));
#63372=CARTESIAN_POINT('Origin',(36.,-5.4,1.75));
#63373=CARTESIAN_POINT('',(36.8,-5.4,1.7));
#63374=CARTESIAN_POINT('Origin',(36.75,-2.7,1.75));
#63375=CARTESIAN_POINT('',(36.8,5.4,1.7));
#63376=CARTESIAN_POINT('Origin',(36.,5.4,1.75));
#63377=CARTESIAN_POINT('',(36.,6.2,1.7));
#63378=CARTESIAN_POINT('Origin',(30.5073223304703,1.35,0.217677669529665));
#63379=CARTESIAN_POINT('',(30.4646446609407,-5.4,0.235355339059329));
#63380=CARTESIAN_POINT('',(30.55,-5.4,0.2));
#63381=CARTESIAN_POINT('',(30.4646446609407,5.4,0.235355339059329));
#63382=CARTESIAN_POINT('',(30.4646446609407,1.35,0.23535533905933));
#63383=CARTESIAN_POINT('',(30.4646446609407,5.4,0.235355339059329));
#63384=CARTESIAN_POINT('Origin',(31.2,-5.4,0.217677669529663));
#63385=CARTESIAN_POINT('',(31.2,-6.13535533905933,0.235355339059327));
#63386=CARTESIAN_POINT('',(31.2,-6.05,0.2));
#63387=CARTESIAN_POINT('Origin',(31.2,-5.4,0.235355339059327));
#63388=CARTESIAN_POINT('Origin',(33.,-6.09267766952966,0.217677669529664));
#63389=CARTESIAN_POINT('',(36.,-6.13535533905933,0.235355339059327));
#63390=CARTESIAN_POINT('',(36.,-6.05,0.2));
#63391=CARTESIAN_POINT('',(33.,-6.13535533905933,0.235355339059327));
#63392=CARTESIAN_POINT('Origin',(36.,-5.4,0.217677669529663));
#63393=CARTESIAN_POINT('',(36.7353553390593,-5.4,0.235355339059329));
#63394=CARTESIAN_POINT('',(36.65,-5.4,0.2));
#63395=CARTESIAN_POINT('Origin',(36.,-5.4,0.235355339059325));
#63396=CARTESIAN_POINT('Origin',(36.6926776695297,-1.35,0.217677669529663));
#63397=CARTESIAN_POINT('',(36.7353553390593,5.4,0.235355339059326));
#63398=CARTESIAN_POINT('',(36.65,5.4,0.2));
#63399=CARTESIAN_POINT('',(36.7353553390593,-1.35,0.235355339059326));
#63400=CARTESIAN_POINT('Origin',(36.,5.4,0.217677669529663));
#63401=CARTESIAN_POINT('',(36.,6.13535533905932,0.235355339059322));
#63402=CARTESIAN_POINT('',(36.,6.04999999999999,0.2));
#63403=CARTESIAN_POINT('Origin',(36.,5.4,0.235355339059326));
#63404=CARTESIAN_POINT('Origin',(34.2,6.09267766952966,0.217677669529664));
#63405=CARTESIAN_POINT('',(31.2,6.13535533905933,0.235355339059327));
#63406=CARTESIAN_POINT('',(31.2,6.05,0.2));
#63407=CARTESIAN_POINT('',(34.2,6.13535533905933,0.235355339059327));
#63408=CARTESIAN_POINT('Origin',(31.2,5.4,0.217677669529663));
#63409=CARTESIAN_POINT('Origin',(31.2,5.4,0.235355339059326));
#63410=CARTESIAN_POINT('Origin',(36.,5.4,0.25));
#63411=CARTESIAN_POINT('',(36.,6.16464466094067,0.264644660940673));
#63412=CARTESIAN_POINT('',(36.,6.1,0.2));
#63413=CARTESIAN_POINT('',(36.7646446609407,5.4,0.264644660940674));
#63414=CARTESIAN_POINT('Origin',(36.,5.4,0.264644660940677));
#63415=CARTESIAN_POINT('',(36.7,5.4,0.2));
#63416=CARTESIAN_POINT('Origin',(34.8,6.15,0.25));
#63417=CARTESIAN_POINT('',(31.2,6.16464466094067,0.264644660940674));
#63418=CARTESIAN_POINT('',(31.2,6.1,0.2));
#63419=CARTESIAN_POINT('',(35.4,6.16464466094067,0.264644660940673));
#63420=CARTESIAN_POINT('Origin',(31.2,5.4,0.25));
#63421=CARTESIAN_POINT('',(30.4353553390593,5.4,0.264644660940674));
#63422=CARTESIAN_POINT('',(30.4,5.4,0.3));
#63423=CARTESIAN_POINT('Origin',(31.2,5.4,0.264644660940674));
#63424=CARTESIAN_POINT('Origin',(30.45,2.7,0.25));
#63425=CARTESIAN_POINT('',(30.4353553390593,-5.4,0.264644660940674));
#63426=CARTESIAN_POINT('',(30.5,-5.4,0.2));
#63427=CARTESIAN_POINT('',(30.4353553390593,4.05,0.264644660940673));
#63428=CARTESIAN_POINT('Origin',(30.4176776695297,4.05,0.307322330470338));
#63429=CARTESIAN_POINT('',(30.4,5.4,0.350000000000003));
#63430=CARTESIAN_POINT('',(30.4353553390593,-5.4,0.264644660940674));
#63431=CARTESIAN_POINT('Origin',(31.2,5.4,0.307322330470338));
#63432=CARTESIAN_POINT('',(31.2,6.2,0.350000000000001));
#63433=CARTESIAN_POINT('Origin',(35.4,6.18232233047034,0.307322330470336));
#63434=CARTESIAN_POINT('',(36.,6.2,0.35));
#63435=CARTESIAN_POINT('Origin',(36.,5.4,0.307322330470339));
#63436=CARTESIAN_POINT('',(36.8,5.4,0.350000000000001));
#63437=CARTESIAN_POINT('Origin',(36.7823223304703,-4.05,0.307322330470338));
#63438=CARTESIAN_POINT('',(36.8,-5.4,0.350000000000001));
#63439=CARTESIAN_POINT('',(36.7646446609407,-5.4,0.264644660940673));
#63440=CARTESIAN_POINT('',(36.8,-5.4,0.350000000000001));
#63441=CARTESIAN_POINT('',(36.7646446609407,-4.05,0.264644660940674));
#63442=CARTESIAN_POINT('',(36.8,-4.05,0.350000000000001));
#63443=CARTESIAN_POINT('Origin',(36.,-5.4,0.307322330470338));
#63444=CARTESIAN_POINT('',(36.,-6.2,0.350000000000001));
#63445=CARTESIAN_POINT('',(36.,-6.16464466094067,0.264644660940674));
#63446=CARTESIAN_POINT('',(36.,-6.2,0.350000000000001));
#63447=CARTESIAN_POINT('Origin',(36.,-5.4,0.264644660940675));
#63448=CARTESIAN_POINT('Origin',(36.,-5.4,0.350000000000001));
#63449=CARTESIAN_POINT('Origin',(31.8,-6.18232233047034,0.307322330470336));
#63450=CARTESIAN_POINT('',(31.2,-6.2,0.35));
#63451=CARTESIAN_POINT('',(31.2,-6.16464466094067,0.264644660940673));
#63452=CARTESIAN_POINT('',(31.2,-6.2,0.35));
#63453=CARTESIAN_POINT('',(31.8,-6.16464466094067,0.264644660940673));
#63454=CARTESIAN_POINT('',(31.8,-6.2,0.35));
#63455=CARTESIAN_POINT('Origin',(31.2,-5.4,0.307322330470338));
#63456=CARTESIAN_POINT('Origin',(31.2,-5.4,0.264644660940674));
#63457=CARTESIAN_POINT('Origin',(31.2,-5.4,0.350000000000002));
#63458=CARTESIAN_POINT('Origin',(36.,-5.4,0.25));
#63459=CARTESIAN_POINT('',(36.7,-5.4,0.2));
#63460=CARTESIAN_POINT('',(36.,-6.1,0.2));
#63461=CARTESIAN_POINT('Origin',(32.4,-6.15,0.25));
#63462=CARTESIAN_POINT('',(31.2,-6.1,0.2));
#63463=CARTESIAN_POINT('Origin',(31.2,-5.4,0.25));
#63464=CARTESIAN_POINT('Origin',(36.75,-2.7,0.25));
#63465=CARTESIAN_POINT('Origin',(30.45,2.7,1.75));
#63466=CARTESIAN_POINT('',(30.4,-5.4,1.7));
#63467=CARTESIAN_POINT('',(30.5,5.4,1.8));
#63468=CARTESIAN_POINT('Origin',(31.2,-5.4,1.75));
#63469=CARTESIAN_POINT('Origin',(34.8,6.15,1.75));
#63470=CARTESIAN_POINT('',(31.2,6.2,1.7));
#63471=CARTESIAN_POINT('Origin',(31.2,5.4,1.75));
#63472=CARTESIAN_POINT('Origin',(36.,-5.4,0.2));
#63473=CARTESIAN_POINT('',(36.,-6.2,0.2));
#63474=CARTESIAN_POINT('',(36.8,-5.4,0.2));
#63475=CARTESIAN_POINT('Origin',(31.2,-6.2,0.2));
#63476=CARTESIAN_POINT('',(31.2,-6.2,0.2));
#63477=CARTESIAN_POINT('Origin',(31.2,-5.4,0.2));
#63478=CARTESIAN_POINT('Origin',(36.8,-5.4,0.2));
#76633=UNCERTAINTY_MEASURE_WITH_UNIT(LENGTH_MEASURE(0.001),#76661,
'DISTANCE_ACCURACY_VALUE',
'Maximum model space distance between geometric entities at asserted c
onnectivities');
#76638=UNCERTAINTY_MEASURE_WITH_UNIT(LENGTH_MEASURE(0.001),#76661,
'DISTANCE_ACCURACY_VALUE',
'Maximum model space distance between geometric entities at asserted c
onnectivities');
#76655=(
GEOMETRIC_REPRESENTATION_CONTEXT(3)
GLOBAL_UNCERTAINTY_ASSIGNED_CONTEXT((#76633))
GLOBAL_UNIT_ASSIGNED_CONTEXT((#76661,#76663,#76664))
REPRESENTATION_CONTEXT('','3D')
);
#76660=(
GEOMETRIC_REPRESENTATION_CONTEXT(3)
GLOBAL_UNCERTAINTY_ASSIGNED_CONTEXT((#76638))
GLOBAL_UNIT_ASSIGNED_CONTEXT((#76661,#76663,#76664))
REPRESENTATION_CONTEXT('','3D')
);
#76661=(
LENGTH_UNIT()
NAMED_UNIT(*)
SI_UNIT(.CENTI.,.METRE.)
);
#76663=(
NAMED_UNIT(*)
PLANE_ANGLE_UNIT()
SI_UNIT($,.RADIAN.)
);
#76664=(
NAMED_UNIT(*)
SI_UNIT($,.STERADIAN.)
SOLID_ANGLE_UNIT()
);
#76681=SHAPE_DEFINITION_REPRESENTATION(#76702,#76751);
#76702=PRODUCT_DEFINITION_SHAPE('',$,#76773);
#76751=SHAPE_REPRESENTATION('',(#28431),#76655);
#76756=PRODUCT_DEFINITION_CONTEXT('part definition',#76821,'design');
#76773=PRODUCT_DEFINITION('2026-10-26-11-13-38-253',
'18_Tailstock_Bed_Clamping_Plate',#76794,#76756);
#76794=PRODUCT_DEFINITION_FORMATION('',$,#76839);
#76821=APPLICATION_CONTEXT(
'Core Data for Automotive Mechanical Design Process');
#76822=PRODUCT_CONTEXT('part definition',#76821,'mechanical');
#76839=PRODUCT('2026-10-26-11-13-38-253',
'18_Tailstock_Bed_Clamping_Plate',$,(#76822));
#76914=COLOUR_RGB('Off White',0.89,0.88,0.83);
#76915=FILL_AREA_STYLE_COLOUR('',#76914);
#76916=FILL_AREA_STYLE('',(#76915));
#76917=SURFACE_STYLE_FILL_AREA(#76916);
#76918=SURFACE_SIDE_STYLE('',(#76917));
#76919=SURFACE_STYLE_USAGE(.BOTH.,#76918);
#76920=PRESENTATION_STYLE_ASSIGNMENT((#76919));
ENDSEC;
END-ISO-10303-21;
